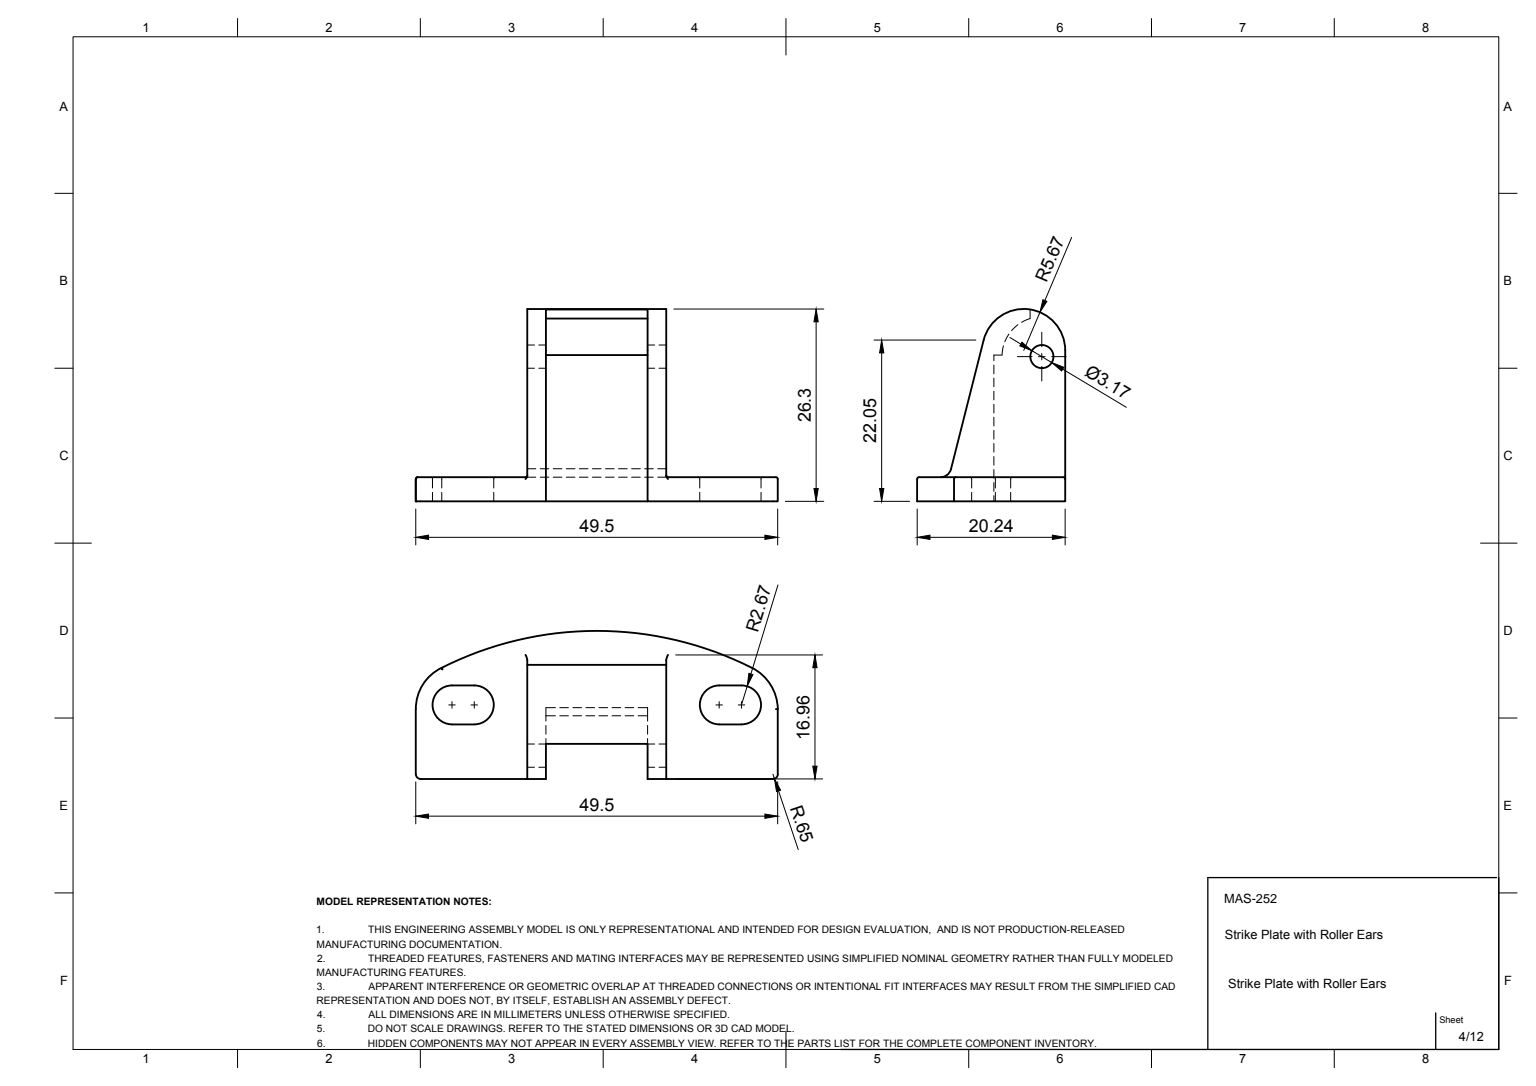
ISO-10303-21;
HEADER;
FILE_DESCRIPTION((''),'2;1');
FILE_NAME('Strike Plate with Roller Ears.step','2026-10-06T07:01:46+05:00',(''),(''),'','','');
FILE_SCHEMA (('AUTOMOTIVE_DESIGN { 1 0 10303 214 3 1 1 }'));
ENDSEC;
DATA;
#10=MECHANICAL_DESIGN_GEOMETRIC_PRESENTATION_REPRESENTATION('',(#139),#11396);
#109=SHAPE_REPRESENTATION_RELATIONSHIP('SRR','None',#11456,#124) ;
#124=ADVANCED_BREP_SHAPE_REPRESENTATION('',(#154),#11382) ;
#139=STYLED_ITEM('',(#11540),#154) ;
#154=MANIFOLD_SOLID_BREP('Strike Plate with Roller Ears',#5570) ;
#191=TOROIDAL_SURFACE('',#5927,0.5,0.25) ;
#192=TOROIDAL_SURFACE('',#5934,0.5,0.25) ;
#193=TOROIDAL_SURFACE('',#5944,2.915,0.25) ;
#194=TOROIDAL_SURFACE('',#5951,2.915,0.25) ;
#195=TOROIDAL_SURFACE('',#5967,2.915,0.25) ;
#196=TOROIDAL_SURFACE('',#5973,2.915,0.25) ;
#197=TOROIDAL_SURFACE('',#5982,5.95626157119474,0.25) ;
#198=TOROIDAL_SURFACE('',#5986,0.399999999999999,0.25) ;
#199=TOROIDAL_SURFACE('',#5990,6.2066222212067,0.25) ;
#200=TOROIDAL_SURFACE('',#5993,46.8573015873016,0.25) ;
#201=TOROIDAL_SURFACE('',#5997,0.400000000000004,0.25) ;
#264=B_SPLINE_CURVE_WITH_KNOTS('',3,(#9098,#9099,#9100,#9101,#9102,#9103,
#9104,#9105,#9106,#9107),.UNSPECIFIED.,.F.,.F.,(4,2,2,2,4),(0.129530190393873,
0.134403051839659,0.157131608255379,0.18177331440849,0.206415020561601),
 .UNSPECIFIED.) ;
#265=B_SPLINE_CURVE_WITH_KNOTS('',3,(#9118,#9119,#9120,#9121,#9122,#9123),
 .UNSPECIFIED.,.F.,.F.,(4,2,4),(0.126383060009627,0.145498866650295,0.174889571433522),
 .UNSPECIFIED.) ;
#266=B_SPLINE_CURVE_WITH_KNOTS('',3,(#9143,#9144,#9145,#9146,#9147,#9148),
 .UNSPECIFIED.,.F.,.F.,(4,2,4),(0.,0.029390704783227,0.0485065114238945),
 .UNSPECIFIED.) ;
#267=B_SPLINE_CURVE_WITH_KNOTS('',3,(#9157,#9158,#9159,#9160,#9161,#9162,
#9163,#9164,#9165,#9166),.UNSPECIFIED.,.F.,.F.,(4,2,2,2,4),(0.176028199507442,
0.200669905660553,0.225311611813664,0.248040168229384,0.252913029669695),
 .UNSPECIFIED.) ;
#268=B_SPLINE_CURVE_WITH_KNOTS('',3,(#9272,#9273,#9274,#9275,#9276,#9277,
#9278,#9279,#9280,#9281,#9282,#9283,#9284,#9285,#9286,#9287,#9288,#9289,
#9290,#9291,#9292,#9293,#9294,#9295,#9296,#9297,#9298,#9299),
 .UNSPECIFIED.,.F.,.F.,(4,3,3,3,3,3,3,3,3,4),(0.,0.196349541608207,0.38455924937953,
0.572733501937903,0.760877527668503,0.94899654600919,1.13718105053103,1.32530713430129,
1.51344881486777,1.57079633286566),.UNSPECIFIED.) ;
#269=B_SPLINE_CURVE_WITH_KNOTS('',3,(#9300,#9301,#9302,#9303,#9304,#9305,
#9306,#9307,#9308,#9309,#9310,#9311),.UNSPECIFIED.,.F.,.F.,(4,2,2,2,2,4),
(-0.0393939259354007,-0.0390590563554235,-0.0292978040547258,-0.0195312295441399,
-0.00976542256445868,0.),.UNSPECIFIED.) ;
#270=B_SPLINE_CURVE_WITH_KNOTS('',3,(#9327,#9328,#9329,#9330,#9331,#9332,
#9333,#9334,#9335,#9336,#9337,#9338),.UNSPECIFIED.,.F.,.F.,(4,2,2,2,2,4),
(-0.000371179043213308,0.,0.00972368624128075,0.0194900624985635,0.0292560287472632,
0.039021789210692),.UNSPECIFIED.) ;
#351=FACE_BOUND('',#949,.T.) ;
#352=FACE_BOUND('',#953,.T.) ;
#353=FACE_BOUND('',#961,.T.) ;
#354=FACE_BOUND('',#962,.T.) ;
#355=FACE_BOUND('',#992,.T.) ;
#356=FACE_BOUND('',#998,.T.) ;
#357=FACE_BOUND('',#1000,.T.) ;
#358=FACE_BOUND('',#1001,.T.) ;
#392=ELLIPSE('',#5926,0.353553390593277,0.25) ;
#393=ELLIPSE('',#5939,0.353553390593277,0.25) ;
#424=PLANE('',#5930) ;
#425=PLANE('',#5940) ;
#426=PLANE('',#5956) ;
#427=PLANE('',#5959) ;
#428=PLANE('',#5977) ;
#429=PLANE('',#6001) ;
#430=PLANE('',#6004) ;
#431=PLANE('',#6011) ;
#432=PLANE('',#6014) ;
#433=PLANE('',#6019) ;
#434=PLANE('',#6022) ;
#435=PLANE('',#6023) ;
#436=PLANE('',#6026) ;
#437=PLANE('',#6027) ;
#438=PLANE('',#6029) ;
#439=PLANE('',#6032) ;
#440=PLANE('',#6034) ;
#441=PLANE('',#6036) ;
#596=FACE_OUTER_BOUND('',#946,.T.) ;
#597=FACE_OUTER_BOUND('',#947,.T.) ;
#598=FACE_OUTER_BOUND('',#948,.T.) ;
#599=FACE_OUTER_BOUND('',#950,.T.) ;
#600=FACE_OUTER_BOUND('',#951,.T.) ;
#601=FACE_OUTER_BOUND('',#952,.T.) ;
#602=FACE_OUTER_BOUND('',#954,.T.) ;
#603=FACE_OUTER_BOUND('',#955,.T.) ;
#604=FACE_OUTER_BOUND('',#956,.T.) ;
#605=FACE_OUTER_BOUND('',#957,.T.) ;
#606=FACE_OUTER_BOUND('',#958,.T.) ;
#607=FACE_OUTER_BOUND('',#959,.T.) ;
#608=FACE_OUTER_BOUND('',#960,.T.) ;
#609=FACE_OUTER_BOUND('',#963,.T.) ;
#610=FACE_OUTER_BOUND('',#964,.T.) ;
#611=FACE_OUTER_BOUND('',#965,.T.) ;
#612=FACE_OUTER_BOUND('',#966,.T.) ;
#613=FACE_OUTER_BOUND('',#967,.T.) ;
#614=FACE_OUTER_BOUND('',#968,.T.) ;
#615=FACE_OUTER_BOUND('',#969,.T.) ;
#616=FACE_OUTER_BOUND('',#970,.T.) ;
#617=FACE_OUTER_BOUND('',#971,.T.) ;
#618=FACE_OUTER_BOUND('',#972,.T.) ;
#619=FACE_OUTER_BOUND('',#973,.T.) ;
#620=FACE_OUTER_BOUND('',#974,.T.) ;
#621=FACE_OUTER_BOUND('',#975,.T.) ;
#622=FACE_OUTER_BOUND('',#976,.T.) ;
#623=FACE_OUTER_BOUND('',#977,.T.) ;
#624=FACE_OUTER_BOUND('',#978,.T.) ;
#625=FACE_OUTER_BOUND('',#979,.T.) ;
#626=FACE_OUTER_BOUND('',#980,.T.) ;
#627=FACE_OUTER_BOUND('',#981,.T.) ;
#628=FACE_OUTER_BOUND('',#982,.T.) ;
#629=FACE_OUTER_BOUND('',#983,.T.) ;
#630=FACE_OUTER_BOUND('',#984,.T.) ;
#631=FACE_OUTER_BOUND('',#985,.T.) ;
#632=FACE_OUTER_BOUND('',#986,.T.) ;
#633=FACE_OUTER_BOUND('',#987,.T.) ;
#634=FACE_OUTER_BOUND('',#988,.T.) ;
#635=FACE_OUTER_BOUND('',#989,.T.) ;
#636=FACE_OUTER_BOUND('',#990,.T.) ;
#637=FACE_OUTER_BOUND('',#991,.T.) ;
#638=FACE_OUTER_BOUND('',#993,.T.) ;
#639=FACE_OUTER_BOUND('',#994,.T.) ;
#640=FACE_OUTER_BOUND('',#995,.T.) ;
#641=FACE_OUTER_BOUND('',#996,.T.) ;
#642=FACE_OUTER_BOUND('',#997,.T.) ;
#643=FACE_OUTER_BOUND('',#999,.T.) ;
#644=FACE_OUTER_BOUND('',#1002,.T.) ;
#645=FACE_OUTER_BOUND('',#1003,.T.) ;
#646=FACE_OUTER_BOUND('',#1004,.T.) ;
#647=FACE_OUTER_BOUND('',#1005,.T.) ;
#648=FACE_OUTER_BOUND('',#1006,.T.) ;
#649=FACE_OUTER_BOUND('',#1007,.T.) ;
#946=EDGE_LOOP('',(#3968,#3969,#3970,#3971,#3972)) ;
#947=EDGE_LOOP('',(#3973,#3974,#3975,#3976)) ;
#948=EDGE_LOOP('',(#3977,#3978,#3979,#3980,#3981,#3982)) ;
#949=EDGE_LOOP('',(#3983)) ;
#950=EDGE_LOOP('',(#3984,#3985,#3986,#3987)) ;
#951=EDGE_LOOP('',(#3988,#3989,#3990,#3991,#3992)) ;
#952=EDGE_LOOP('',(#3993,#3994,#3995,#3996,#3997,#3998)) ;
#953=EDGE_LOOP('',(#3999)) ;
#954=EDGE_LOOP('',(#4000,#4001,#4002,#4003)) ;
#955=EDGE_LOOP('',(#4004,#4005,#4006,#4007)) ;
#956=EDGE_LOOP('',(#4008,#4009,#4010,#4011)) ;
#957=EDGE_LOOP('',(#4012,#4013,#4014,#4015)) ;
#958=EDGE_LOOP('',(#4016,#4017,#4018,#4019)) ;
#959=EDGE_LOOP('',(#4020,#4021,#4022,#4023)) ;
#960=EDGE_LOOP('',(#4024,#4025,#4026,#4027,#4028,#4029,#4030,#4031,#4032,
#4033,#4034,#4035)) ;
#961=EDGE_LOOP('',(#4036,#4037,#4038,#4039)) ;
#962=EDGE_LOOP('',(#4040,#4041,#4042,#4043)) ;
#963=EDGE_LOOP('',(#4044,#4045,#4046,#4047)) ;
#964=EDGE_LOOP('',(#4048,#4049,#4050,#4051)) ;
#965=EDGE_LOOP('',(#4052,#4053,#4054,#4055)) ;
#966=EDGE_LOOP('',(#4056,#4057,#4058,#4059)) ;
#967=EDGE_LOOP('',(#4060,#4061,#4062,#4063)) ;
#968=EDGE_LOOP('',(#4064,#4065,#4066,#4067)) ;
#969=EDGE_LOOP('',(#4068,#4069,#4070,#4071)) ;
#970=EDGE_LOOP('',(#4072,#4073,#4074,#4075,#4076,#4077)) ;
#971=EDGE_LOOP('',(#4078,#4079,#4080,#4081)) ;
#972=EDGE_LOOP('',(#4082,#4083,#4084,#4085)) ;
#973=EDGE_LOOP('',(#4086,#4087,#4088,#4089)) ;
#974=EDGE_LOOP('',(#4090,#4091,#4092,#4093)) ;
#975=EDGE_LOOP('',(#4094,#4095,#4096,#4097)) ;
#976=EDGE_LOOP('',(#4098,#4099,#4100,#4101)) ;
#977=EDGE_LOOP('',(#4102,#4103,#4104,#4105)) ;
#978=EDGE_LOOP('',(#4106,#4107,#4108,#4109)) ;
#979=EDGE_LOOP('',(#4110,#4111,#4112,#4113)) ;
#980=EDGE_LOOP('',(#4114,#4115,#4116,#4117,#4118,#4119,#4120)) ;
#981=EDGE_LOOP('',(#4121,#4122,#4123,#4124)) ;
#982=EDGE_LOOP('',(#4125,#4126,#4127,#4128)) ;
#983=EDGE_LOOP('',(#4129,#4130,#4131,#4132)) ;
#984=EDGE_LOOP('',(#4133,#4134,#4135,#4136)) ;
#985=EDGE_LOOP('',(#4137,#4138,#4139,#4140)) ;
#986=EDGE_LOOP('',(#4141,#4142,#4143,#4144)) ;
#987=EDGE_LOOP('',(#4145,#4146,#4147,#4148)) ;
#988=EDGE_LOOP('',(#4149,#4150,#4151,#4152,#4153,#4154,#4155)) ;
#989=EDGE_LOOP('',(#4156,#4157,#4158,#4159)) ;
#990=EDGE_LOOP('',(#4160,#4161,#4162,#4163)) ;
#991=EDGE_LOOP('',(#4164,#4165,#4166,#4167,#4168,#4169,#4170)) ;
#992=EDGE_LOOP('',(#4171)) ;
#993=EDGE_LOOP('',(#4172,#4173,#4174,#4175)) ;
#994=EDGE_LOOP('',(#4176,#4177,#4178,#4179)) ;
#995=EDGE_LOOP('',(#4180,#4181,#4182,#4183)) ;
#996=EDGE_LOOP('',(#4184,#4185,#4186,#4187)) ;
#997=EDGE_LOOP('',(#4188,#4189,#4190,#4191,#4192,#4193,#4194)) ;
#998=EDGE_LOOP('',(#4195)) ;
#999=EDGE_LOOP('',(#4196,#4197,#4198,#4199,#4200,#4201,#4202,#4203,#4204,
#4205,#4206,#4207)) ;
#1000=EDGE_LOOP('',(#4208,#4209,#4210,#4211)) ;
#1001=EDGE_LOOP('',(#4212,#4213,#4214,#4215)) ;
#1002=EDGE_LOOP('',(#4216,#4217,#4218,#4219)) ;
#1003=EDGE_LOOP('',(#4220,#4221,#4222,#4223,#4224,#4225,#4226,#4227)) ;
#1004=EDGE_LOOP('',(#4228,#4229,#4230,#4231)) ;
#1005=EDGE_LOOP('',(#4232,#4233,#4234,#4235)) ;
#1006=EDGE_LOOP('',(#4236,#4237,#4238,#4239)) ;
#1007=EDGE_LOOP('',(#4240,#4241,#4242,#4243)) ;
#1326=LINE('',#9109,#1709) ;
#1327=LINE('',#9113,#1710) ;
#1328=LINE('',#9130,#1711) ;
#1329=LINE('',#9133,#1712) ;
#1330=LINE('',#9154,#1713) ;
#1331=LINE('',#9156,#1714) ;
#1332=LINE('',#9169,#1715) ;
#1333=LINE('',#9173,#1716) ;
#1334=LINE('',#9190,#1717) ;
#1335=LINE('',#9191,#1718) ;
#1336=LINE('',#9199,#1719) ;
#1337=LINE('',#9200,#1720) ;
#1338=LINE('',#9203,#1721) ;
#1339=LINE('',#9205,#1722) ;
#1340=LINE('',#9206,#1723) ;
#1341=LINE('',#9209,#1724) ;
#1342=LINE('',#9213,#1725) ;
#1343=LINE('',#9217,#1726) ;
#1344=LINE('',#9225,#1727) ;
#1345=LINE('',#9228,#1728) ;
#1346=LINE('',#9229,#1729) ;
#1347=LINE('',#9234,#1730) ;
#1348=LINE('',#9237,#1731) ;
#1349=LINE('',#9247,#1732) ;
#1350=LINE('',#9253,#1733) ;
#1351=LINE('',#9256,#1734) ;
#1352=LINE('',#9258,#1735) ;
#1353=LINE('',#9259,#1736) ;
#1354=LINE('',#9262,#1737) ;
#1355=LINE('',#9265,#1738) ;
#1356=LINE('',#9267,#1739) ;
#1357=LINE('',#9314,#1740) ;
#1358=LINE('',#9321,#1741) ;
#1359=LINE('',#9343,#1742) ;
#1360=LINE('',#9350,#1743) ;
#1361=LINE('',#9353,#1744) ;
#1362=LINE('',#9355,#1745) ;
#1363=LINE('',#9357,#1746) ;
#1364=LINE('',#9358,#1747) ;
#1365=LINE('',#9361,#1748) ;
#1366=LINE('',#9365,#1749) ;
#1367=LINE('',#9366,#1750) ;
#1368=LINE('',#9369,#1751) ;
#1369=LINE('',#9373,#1752) ;
#1370=LINE('',#9377,#1753) ;
#1371=LINE('',#9381,#1754) ;
#1372=LINE('',#9382,#1755) ;
#1373=LINE('',#9385,#1756) ;
#1374=LINE('',#9389,#1757) ;
#1375=LINE('',#9391,#1758) ;
#1376=LINE('',#9392,#1759) ;
#1377=LINE('',#9395,#1760) ;
#1378=LINE('',#9400,#1761) ;
#1379=LINE('',#9403,#1762) ;
#1380=LINE('',#9405,#1763) ;
#1381=LINE('',#9407,#1764) ;
#1382=LINE('',#9411,#1765) ;
#1383=LINE('',#9416,#1766) ;
#1384=LINE('',#9417,#1767) ;
#1385=LINE('',#9418,#1768) ;
#1386=LINE('',#9421,#1769) ;
#1387=LINE('',#9422,#1770) ;
#1388=LINE('',#9426,#1771) ;
#1389=LINE('',#9429,#1772) ;
#1390=LINE('',#9430,#1773) ;
#1391=LINE('',#9433,#1774) ;
#1392=LINE('',#9436,#1775) ;
#1393=LINE('',#9439,#1776) ;
#1394=LINE('',#9442,#1777) ;
#1395=LINE('',#9445,#1778) ;
#1396=LINE('',#9448,#1779) ;
#1709=VECTOR('',#6870,10.) ;
#1710=VECTOR('',#6873,10.) ;
#1711=VECTOR('',#6886,10.) ;
#1712=VECTOR('',#6889,10.) ;
#1713=VECTOR('',#6904,10.) ;
#1714=VECTOR('',#6905,10.) ;
#1715=VECTOR('',#6908,10.) ;
#1716=VECTOR('',#6911,10.) ;
#1717=VECTOR('',#6930,10.) ;
#1718=VECTOR('',#6931,10.) ;
#1719=VECTOR('',#6942,10.) ;
#1720=VECTOR('',#6943,10.) ;
#1721=VECTOR('',#6946,10.) ;
#1722=VECTOR('',#6947,10.) ;
#1723=VECTOR('',#6948,10.) ;
#1724=VECTOR('',#6951,10.) ;
#1725=VECTOR('',#6956,10.) ;
#1726=VECTOR('',#6959,10.) ;
#1727=VECTOR('',#6966,10.) ;
#1728=VECTOR('',#6969,10.) ;
#1729=VECTOR('',#6970,10.) ;
#1730=VECTOR('',#6973,10.) ;
#1731=VECTOR('',#6976,10.) ;
#1732=VECTOR('',#6989,10.) ;
#1733=VECTOR('',#6998,10.) ;
#1734=VECTOR('',#7001,10.) ;
#1735=VECTOR('',#7002,10.) ;
#1736=VECTOR('',#7003,10.) ;
#1737=VECTOR('',#7006,10.) ;
#1738=VECTOR('',#7011,10.) ;
#1739=VECTOR('',#7014,10.) ;
#1740=VECTOR('',#7021,10.) ;
#1741=VECTOR('',#7032,10.) ;
#1742=VECTOR('',#7045,10.) ;
#1743=VECTOR('',#7056,10.) ;
#1744=VECTOR('',#7059,10.) ;
#1745=VECTOR('',#7060,10.) ;
#1746=VECTOR('',#7061,10.) ;
#1747=VECTOR('',#7062,10.) ;
#1748=VECTOR('',#7065,10.) ;
#1749=VECTOR('',#7070,10.) ;
#1750=VECTOR('',#7071,10.) ;
#1751=VECTOR('',#7074,10.) ;
#1752=VECTOR('',#7079,10.) ;
#1753=VECTOR('',#7084,10.) ;
#1754=VECTOR('',#7089,10.) ;
#1755=VECTOR('',#7090,10.) ;
#1756=VECTOR('',#7093,10.) ;
#1757=VECTOR('',#7098,10.) ;
#1758=VECTOR('',#7099,10.) ;
#1759=VECTOR('',#7100,10.) ;
#1760=VECTOR('',#7103,1.585) ;
#1761=VECTOR('',#7110,1.585) ;
#1762=VECTOR('',#7113,10.) ;
#1763=VECTOR('',#7114,10.) ;
#1764=VECTOR('',#7115,10.) ;
#1765=VECTOR('',#7118,10.) ;
#1766=VECTOR('',#7123,10.) ;
#1767=VECTOR('',#7124,10.) ;
#1768=VECTOR('',#7125,10.) ;
#1769=VECTOR('',#7128,10.) ;
#1770=VECTOR('',#7129,10.) ;
#1771=VECTOR('',#7134,10.) ;
#1772=VECTOR('',#7137,10.) ;
#1773=VECTOR('',#7138,10.) ;
#1774=VECTOR('',#7143,10.) ;
#1775=VECTOR('',#7146,10.) ;
#1776=VECTOR('',#7149,10.) ;
#1777=VECTOR('',#7154,10.) ;
#1778=VECTOR('',#7159,10.) ;
#1779=VECTOR('',#7164,10.) ;
#2062=CIRCLE('',#5925,0.25) ;
#2063=CIRCLE('',#5928,0.25) ;
#2064=CIRCLE('',#5929,0.5) ;
#2065=CIRCLE('',#5931,1.48867477559092) ;
#2066=CIRCLE('',#5932,5.66550083849775) ;
#2067=CIRCLE('',#5933,1.585) ;
#2068=CIRCLE('',#5935,0.25) ;
#2069=CIRCLE('',#5936,0.25) ;
#2070=CIRCLE('',#5937,0.5) ;
#2071=CIRCLE('',#5941,5.66550083849775) ;
#2072=CIRCLE('',#5942,1.48867477559092) ;
#2073=CIRCLE('',#5943,1.585) ;
#2074=CIRCLE('',#5945,0.25) ;
#2075=CIRCLE('',#5946,2.665) ;
#2076=CIRCLE('',#5947,0.250000000000004) ;
#2077=CIRCLE('',#5948,2.915) ;
#2078=CIRCLE('',#5950,0.250000000000004) ;
#2079=CIRCLE('',#5952,0.250000000000004) ;
#2080=CIRCLE('',#5953,2.915) ;
#2081=CIRCLE('',#5954,2.665) ;
#2082=CIRCLE('',#5958,2.665) ;
#2083=CIRCLE('',#5960,0.400000000000004) ;
#2084=CIRCLE('',#5961,6.2066222212067) ;
#2085=CIRCLE('',#5962,46.8573015873016) ;
#2086=CIRCLE('',#5963,5.95626157119474) ;
#2087=CIRCLE('',#5964,0.399999999999999) ;
#2088=CIRCLE('',#5965,2.915) ;
#2089=CIRCLE('',#5966,2.915) ;
#2090=CIRCLE('',#5968,0.25) ;
#2091=CIRCLE('',#5969,2.665) ;
#2092=CIRCLE('',#5970,0.250000000000004) ;
#2093=CIRCLE('',#5972,0.250000000000004) ;
#2094=CIRCLE('',#5974,0.250000000000004) ;
#2095=CIRCLE('',#5975,2.665) ;
#2096=CIRCLE('',#5979,2.665) ;
#2097=CIRCLE('',#5983,6.20626157119474) ;
#2098=CIRCLE('',#5985,0.249999999999999) ;
#2099=CIRCLE('',#5987,0.250000000000004) ;
#2100=CIRCLE('',#5988,0.649999999999999) ;
#2101=CIRCLE('',#5991,6.4566222212067) ;
#2102=CIRCLE('',#5992,0.249999999999994) ;
#2103=CIRCLE('',#5994,47.1073015873016) ;
#2104=CIRCLE('',#5996,0.249999999999999) ;
#2105=CIRCLE('',#5998,0.249999999999999) ;
#2106=CIRCLE('',#5999,0.650000000000004) ;
#2107=CIRCLE('',#6003,0.649999999999999) ;
#2108=CIRCLE('',#6006,6.20626157119473) ;
#2109=CIRCLE('',#6008,47.1073015873016) ;
#2110=CIRCLE('',#6010,6.4566222212067) ;
#2111=CIRCLE('',#6013,0.650000000000004) ;
#2112=CIRCLE('',#6016,1.585) ;
#2113=CIRCLE('',#6018,1.585) ;
#2114=CIRCLE('',#6020,5.45) ;
#2115=CIRCLE('',#6021,5.66550083849775) ;
#2116=CIRCLE('',#6025,5.45) ;
#2117=CIRCLE('',#6028,5.66550083849775) ;
#2118=CIRCLE('',#6030,2.665) ;
#2119=CIRCLE('',#6031,2.665) ;
#2403=VERTEX_POINT('',#9096) ;
#2404=VERTEX_POINT('',#9097) ;
#2405=VERTEX_POINT('',#9108) ;
#2406=VERTEX_POINT('',#9110) ;
#2407=VERTEX_POINT('',#9112) ;
#2408=VERTEX_POINT('',#9116) ;
#2409=VERTEX_POINT('',#9117) ;
#2410=VERTEX_POINT('',#9127) ;
#2411=VERTEX_POINT('',#9129) ;
#2412=VERTEX_POINT('',#9131) ;
#2413=VERTEX_POINT('',#9134) ;
#2414=VERTEX_POINT('',#9137) ;
#2415=VERTEX_POINT('',#9138) ;
#2416=VERTEX_POINT('',#9140) ;
#2417=VERTEX_POINT('',#9142) ;
#2418=VERTEX_POINT('',#9151) ;
#2419=VERTEX_POINT('',#9152) ;
#2420=VERTEX_POINT('',#9155) ;
#2421=VERTEX_POINT('',#9168) ;
#2422=VERTEX_POINT('',#9170) ;
#2423=VERTEX_POINT('',#9172) ;
#2424=VERTEX_POINT('',#9175) ;
#2425=VERTEX_POINT('',#9178) ;
#2426=VERTEX_POINT('',#9179) ;
#2427=VERTEX_POINT('',#9181) ;
#2428=VERTEX_POINT('',#9183) ;
#2429=VERTEX_POINT('',#9187) ;
#2430=VERTEX_POINT('',#9188) ;
#2431=VERTEX_POINT('',#9193) ;
#2432=VERTEX_POINT('',#9194) ;
#2433=VERTEX_POINT('',#9202) ;
#2434=VERTEX_POINT('',#9204) ;
#2435=VERTEX_POINT('',#9208) ;
#2436=VERTEX_POINT('',#9212) ;
#2437=VERTEX_POINT('',#9214) ;
#2438=VERTEX_POINT('',#9216) ;
#2439=VERTEX_POINT('',#9218) ;
#2440=VERTEX_POINT('',#9220) ;
#2441=VERTEX_POINT('',#9222) ;
#2442=VERTEX_POINT('',#9224) ;
#2443=VERTEX_POINT('',#9226) ;
#2444=VERTEX_POINT('',#9230) ;
#2445=VERTEX_POINT('',#9231) ;
#2446=VERTEX_POINT('',#9233) ;
#2447=VERTEX_POINT('',#9235) ;
#2448=VERTEX_POINT('',#9239) ;
#2449=VERTEX_POINT('',#9241) ;
#2450=VERTEX_POINT('',#9245) ;
#2451=VERTEX_POINT('',#9249) ;
#2452=VERTEX_POINT('',#9255) ;
#2453=VERTEX_POINT('',#9257) ;
#2454=VERTEX_POINT('',#9261) ;
#2455=VERTEX_POINT('',#9269) ;
#2456=VERTEX_POINT('',#9270) ;
#2457=VERTEX_POINT('',#9313) ;
#2458=VERTEX_POINT('',#9317) ;
#2459=VERTEX_POINT('',#9323) ;
#2460=VERTEX_POINT('',#9324) ;
#2461=VERTEX_POINT('',#9342) ;
#2462=VERTEX_POINT('',#9346) ;
#2463=VERTEX_POINT('',#9352) ;
#2464=VERTEX_POINT('',#9354) ;
#2465=VERTEX_POINT('',#9356) ;
#2466=VERTEX_POINT('',#9360) ;
#2467=VERTEX_POINT('',#9364) ;
#2468=VERTEX_POINT('',#9368) ;
#2469=VERTEX_POINT('',#9372) ;
#2470=VERTEX_POINT('',#9376) ;
#2471=VERTEX_POINT('',#9380) ;
#2472=VERTEX_POINT('',#9384) ;
#2473=VERTEX_POINT('',#9388) ;
#2474=VERTEX_POINT('',#9390) ;
#2475=VERTEX_POINT('',#9394) ;
#2476=VERTEX_POINT('',#9398) ;
#2477=VERTEX_POINT('',#9402) ;
#2478=VERTEX_POINT('',#9404) ;
#2479=VERTEX_POINT('',#9406) ;
#2480=VERTEX_POINT('',#9408) ;
#2481=VERTEX_POINT('',#9410) ;
#2482=VERTEX_POINT('',#9414) ;
#2483=VERTEX_POINT('',#9415) ;
#2484=VERTEX_POINT('',#9420) ;
#2485=VERTEX_POINT('',#9424) ;
#2486=VERTEX_POINT('',#9428) ;
#2487=VERTEX_POINT('',#9435) ;
#2488=VERTEX_POINT('',#9438) ;
#2966=EDGE_CURVE('',#2403,#2404,#264,.T.) ;
#2967=EDGE_CURVE('',#2404,#2405,#1326,.T.) ;
#2968=EDGE_CURVE('',#2405,#2406,#2062,.T.) ;
#2969=EDGE_CURVE('',#2406,#2407,#1327,.T.) ;
#2970=EDGE_CURVE('',#2407,#2403,#392,.T.) ;
#2971=EDGE_CURVE('',#2408,#2409,#265,.T.) ;
#2972=EDGE_CURVE('',#2409,#2406,#2063,.T.) ;
#2973=EDGE_CURVE('',#2405,#2408,#2064,.T.) ;
#2974=EDGE_CURVE('',#2404,#2410,#2065,.T.) ;
#2975=EDGE_CURVE('',#2411,#2410,#1328,.T.) ;
#2976=EDGE_CURVE('',#2412,#2411,#2066,.T.) ;
#2977=EDGE_CURVE('',#2408,#2412,#1329,.T.) ;
#2978=EDGE_CURVE('',#2413,#2413,#2067,.T.) ;
#2979=EDGE_CURVE('',#2414,#2415,#2068,.T.) ;
#2980=EDGE_CURVE('',#2415,#2416,#2069,.T.) ;
#2981=EDGE_CURVE('',#2416,#2417,#266,.T.) ;
#2982=EDGE_CURVE('',#2417,#2414,#2070,.T.) ;
#2983=EDGE_CURVE('',#2418,#2419,#393,.F.) ;
#2984=EDGE_CURVE('',#2418,#2415,#1330,.T.) ;
#2985=EDGE_CURVE('',#2414,#2420,#1331,.T.) ;
#2986=EDGE_CURVE('',#2419,#2420,#267,.F.) ;
#2987=EDGE_CURVE('',#2417,#2421,#1332,.T.) ;
#2988=EDGE_CURVE('',#2421,#2422,#2071,.T.) ;
#2989=EDGE_CURVE('',#2422,#2423,#1333,.T.) ;
#2990=EDGE_CURVE('',#2423,#2420,#2072,.T.) ;
#2991=EDGE_CURVE('',#2424,#2424,#2073,.T.) ;
#2992=EDGE_CURVE('',#2425,#2426,#2074,.T.) ;
#2993=EDGE_CURVE('',#2426,#2427,#2075,.T.) ;
#2994=EDGE_CURVE('',#2427,#2428,#2076,.T.) ;
#2995=EDGE_CURVE('',#2428,#2425,#2077,.T.) ;
#2996=EDGE_CURVE('',#2429,#2430,#2078,.T.) ;
#2997=EDGE_CURVE('',#2430,#2428,#1334,.T.) ;
#2998=EDGE_CURVE('',#2427,#2429,#1335,.T.) ;
#2999=EDGE_CURVE('',#2431,#2432,#2079,.T.) ;
#3000=EDGE_CURVE('',#2432,#2430,#2080,.T.) ;
#3001=EDGE_CURVE('',#2429,#2431,#2081,.T.) ;
#3002=EDGE_CURVE('',#2425,#2432,#1336,.T.) ;
#3003=EDGE_CURVE('',#2431,#2426,#1337,.T.) ;
#3004=EDGE_CURVE('',#2433,#2427,#1338,.T.) ;
#3005=EDGE_CURVE('',#2433,#2434,#1339,.T.) ;
#3006=EDGE_CURVE('',#2434,#2429,#1340,.T.) ;
#3007=EDGE_CURVE('',#2435,#2426,#1341,.T.) ;
#3008=EDGE_CURVE('',#2435,#2433,#2082,.T.) ;
#3009=EDGE_CURVE('',#2436,#2406,#1342,.T.) ;
#3010=EDGE_CURVE('',#2437,#2436,#2083,.T.) ;
#3011=EDGE_CURVE('',#2438,#2437,#1343,.T.) ;
#3012=EDGE_CURVE('',#2439,#2438,#2084,.T.) ;
#3013=EDGE_CURVE('',#2440,#2439,#2085,.T.) ;
#3014=EDGE_CURVE('',#2441,#2440,#2086,.T.) ;
#3015=EDGE_CURVE('',#2442,#2441,#1344,.T.) ;
#3016=EDGE_CURVE('',#2443,#2442,#2087,.T.) ;
#3017=EDGE_CURVE('',#2415,#2443,#1345,.T.) ;
#3018=EDGE_CURVE('',#2407,#2418,#1346,.T.) ;
#3019=EDGE_CURVE('',#2444,#2445,#2088,.T.) ;
#3020=EDGE_CURVE('',#2446,#2444,#1347,.T.) ;
#3021=EDGE_CURVE('',#2447,#2446,#2089,.T.) ;
#3022=EDGE_CURVE('',#2445,#2447,#1348,.T.) ;
#3023=EDGE_CURVE('',#2445,#2448,#2090,.T.) ;
#3024=EDGE_CURVE('',#2448,#2449,#2091,.T.) ;
#3025=EDGE_CURVE('',#2449,#2444,#2092,.T.) ;
#3026=EDGE_CURVE('',#2450,#2446,#2093,.T.) ;
#3027=EDGE_CURVE('',#2449,#2450,#1349,.T.) ;
#3028=EDGE_CURVE('',#2451,#2447,#2094,.T.) ;
#3029=EDGE_CURVE('',#2450,#2451,#2095,.T.) ;
#3030=EDGE_CURVE('',#2451,#2448,#1350,.T.) ;
#3031=EDGE_CURVE('',#2452,#2449,#1351,.T.) ;
#3032=EDGE_CURVE('',#2452,#2453,#1352,.T.) ;
#3033=EDGE_CURVE('',#2453,#2450,#1353,.T.) ;
#3034=EDGE_CURVE('',#2454,#2448,#1354,.T.) ;
#3035=EDGE_CURVE('',#2454,#2452,#2096,.T.) ;
#3036=EDGE_CURVE('',#2419,#2403,#1355,.T.) ;
#3037=EDGE_CURVE('',#2410,#2423,#1356,.T.) ;
#3038=EDGE_CURVE('',#2455,#2456,#2097,.T.) ;
#3039=EDGE_CURVE('',#2456,#2441,#268,.T.) ;
#3040=EDGE_CURVE('',#2440,#2455,#269,.T.) ;
#3041=EDGE_CURVE('',#2456,#2457,#1357,.T.) ;
#3042=EDGE_CURVE('',#2457,#2442,#2098,.T.) ;
#3043=EDGE_CURVE('',#2458,#2443,#2099,.T.) ;
#3044=EDGE_CURVE('',#2457,#2458,#2100,.T.) ;
#3045=EDGE_CURVE('',#2458,#2416,#1358,.T.) ;
#3046=EDGE_CURVE('',#2459,#2460,#2101,.T.) ;
#3047=EDGE_CURVE('',#2460,#2439,#2102,.T.) ;
#3048=EDGE_CURVE('',#2438,#2459,#270,.T.) ;
#3049=EDGE_CURVE('',#2460,#2455,#2103,.T.) ;
#3050=EDGE_CURVE('',#2409,#2461,#1359,.T.) ;
#3051=EDGE_CURVE('',#2461,#2436,#2104,.T.) ;
#3052=EDGE_CURVE('',#2462,#2437,#2105,.T.) ;
#3053=EDGE_CURVE('',#2461,#2462,#2106,.T.) ;
#3054=EDGE_CURVE('',#2462,#2459,#1360,.T.) ;
#3055=EDGE_CURVE('',#2463,#2458,#1361,.T.) ;
#3056=EDGE_CURVE('',#2464,#2463,#1362,.T.) ;
#3057=EDGE_CURVE('',#2464,#2465,#1363,.T.) ;
#3058=EDGE_CURVE('',#2465,#2421,#1364,.T.) ;
#3059=EDGE_CURVE('',#2466,#2457,#1365,.T.) ;
#3060=EDGE_CURVE('',#2466,#2463,#2107,.T.) ;
#3061=EDGE_CURVE('',#2467,#2456,#1366,.T.) ;
#3062=EDGE_CURVE('',#2466,#2467,#1367,.T.) ;
#3063=EDGE_CURVE('',#2468,#2455,#1368,.T.) ;
#3064=EDGE_CURVE('',#2468,#2467,#2108,.T.) ;
#3065=EDGE_CURVE('',#2469,#2460,#1369,.T.) ;
#3066=EDGE_CURVE('',#2469,#2468,#2109,.T.) ;
#3067=EDGE_CURVE('',#2470,#2459,#1370,.T.) ;
#3068=EDGE_CURVE('',#2470,#2469,#2110,.T.) ;
#3069=EDGE_CURVE('',#2471,#2462,#1371,.T.) ;
#3070=EDGE_CURVE('',#2470,#2471,#1372,.T.) ;
#3071=EDGE_CURVE('',#2472,#2461,#1373,.T.) ;
#3072=EDGE_CURVE('',#2472,#2471,#2111,.T.) ;
#3073=EDGE_CURVE('',#2412,#2473,#1374,.T.) ;
#3074=EDGE_CURVE('',#2473,#2474,#1375,.T.) ;
#3075=EDGE_CURVE('',#2472,#2474,#1376,.T.) ;
#3076=EDGE_CURVE('',#2413,#2475,#1377,.T.) ;
#3077=EDGE_CURVE('',#2475,#2475,#2112,.T.) ;
#3078=EDGE_CURVE('',#2476,#2476,#2113,.T.) ;
#3079=EDGE_CURVE('',#2476,#2424,#1378,.T.) ;
#3080=EDGE_CURVE('',#2477,#2464,#1379,.T.) ;
#3081=EDGE_CURVE('',#2478,#2477,#1380,.T.) ;
#3082=EDGE_CURVE('',#2479,#2478,#1381,.T.) ;
#3083=EDGE_CURVE('',#2480,#2479,#2114,.T.) ;
#3084=EDGE_CURVE('',#2481,#2480,#1382,.T.) ;
#3085=EDGE_CURVE('',#2465,#2481,#2115,.T.) ;
#3086=EDGE_CURVE('',#2482,#2483,#1383,.T.) ;
#3087=EDGE_CURVE('',#2482,#2478,#1384,.T.) ;
#3088=EDGE_CURVE('',#2483,#2477,#1385,.T.) ;
#3089=EDGE_CURVE('',#2484,#2482,#1386,.T.) ;
#3090=EDGE_CURVE('',#2484,#2479,#1387,.T.) ;
#3091=EDGE_CURVE('',#2485,#2484,#2116,.T.) ;
#3092=EDGE_CURVE('',#2485,#2480,#1388,.T.) ;
#3093=EDGE_CURVE('',#2481,#2486,#1389,.T.) ;
#3094=EDGE_CURVE('',#2486,#2485,#1390,.T.) ;
#3095=EDGE_CURVE('',#2486,#2473,#2117,.T.) ;
#3096=EDGE_CURVE('',#2474,#2483,#1391,.T.) ;
#3097=EDGE_CURVE('',#2487,#2454,#1392,.T.) ;
#3098=EDGE_CURVE('',#2453,#2487,#2118,.T.) ;
#3099=EDGE_CURVE('',#2488,#2435,#1393,.T.) ;
#3100=EDGE_CURVE('',#2434,#2488,#2119,.T.) ;
#3101=EDGE_CURVE('',#2411,#2422,#1394,.T.) ;
#3102=EDGE_CURVE('',#2487,#2451,#1395,.T.) ;
#3103=EDGE_CURVE('',#2488,#2431,#1396,.T.) ;
#3968=ORIENTED_EDGE('',*,*,#2966,.T.) ;
#3969=ORIENTED_EDGE('',*,*,#2967,.T.) ;
#3970=ORIENTED_EDGE('',*,*,#2968,.T.) ;
#3971=ORIENTED_EDGE('',*,*,#2969,.T.) ;
#3972=ORIENTED_EDGE('',*,*,#2970,.T.) ;
#3973=ORIENTED_EDGE('',*,*,#2971,.T.) ;
#3974=ORIENTED_EDGE('',*,*,#2972,.T.) ;
#3975=ORIENTED_EDGE('',*,*,#2968,.F.) ;
#3976=ORIENTED_EDGE('',*,*,#2973,.T.) ;
#3977=ORIENTED_EDGE('',*,*,#2973,.F.) ;
#3978=ORIENTED_EDGE('',*,*,#2967,.F.) ;
#3979=ORIENTED_EDGE('',*,*,#2974,.T.) ;
#3980=ORIENTED_EDGE('',*,*,#2975,.F.) ;
#3981=ORIENTED_EDGE('',*,*,#2976,.F.) ;
#3982=ORIENTED_EDGE('',*,*,#2977,.F.) ;
#3983=ORIENTED_EDGE('',*,*,#2978,.T.) ;
#3984=ORIENTED_EDGE('',*,*,#2979,.T.) ;
#3985=ORIENTED_EDGE('',*,*,#2980,.T.) ;
#3986=ORIENTED_EDGE('',*,*,#2981,.T.) ;
#3987=ORIENTED_EDGE('',*,*,#2982,.T.) ;
#3988=ORIENTED_EDGE('',*,*,#2983,.F.) ;
#3989=ORIENTED_EDGE('',*,*,#2984,.T.) ;
#3990=ORIENTED_EDGE('',*,*,#2979,.F.) ;
#3991=ORIENTED_EDGE('',*,*,#2985,.T.) ;
#3992=ORIENTED_EDGE('',*,*,#2986,.F.) ;
#3993=ORIENTED_EDGE('',*,*,#2985,.F.) ;
#3994=ORIENTED_EDGE('',*,*,#2982,.F.) ;
#3995=ORIENTED_EDGE('',*,*,#2987,.T.) ;
#3996=ORIENTED_EDGE('',*,*,#2988,.T.) ;
#3997=ORIENTED_EDGE('',*,*,#2989,.T.) ;
#3998=ORIENTED_EDGE('',*,*,#2990,.T.) ;
#3999=ORIENTED_EDGE('',*,*,#2991,.T.) ;
#4000=ORIENTED_EDGE('',*,*,#2992,.T.) ;
#4001=ORIENTED_EDGE('',*,*,#2993,.T.) ;
#4002=ORIENTED_EDGE('',*,*,#2994,.T.) ;
#4003=ORIENTED_EDGE('',*,*,#2995,.T.) ;
#4004=ORIENTED_EDGE('',*,*,#2996,.T.) ;
#4005=ORIENTED_EDGE('',*,*,#2997,.T.) ;
#4006=ORIENTED_EDGE('',*,*,#2994,.F.) ;
#4007=ORIENTED_EDGE('',*,*,#2998,.T.) ;
#4008=ORIENTED_EDGE('',*,*,#2999,.T.) ;
#4009=ORIENTED_EDGE('',*,*,#3000,.T.) ;
#4010=ORIENTED_EDGE('',*,*,#2996,.F.) ;
#4011=ORIENTED_EDGE('',*,*,#3001,.T.) ;
#4012=ORIENTED_EDGE('',*,*,#2992,.F.) ;
#4013=ORIENTED_EDGE('',*,*,#3002,.T.) ;
#4014=ORIENTED_EDGE('',*,*,#2999,.F.) ;
#4015=ORIENTED_EDGE('',*,*,#3003,.T.) ;
#4016=ORIENTED_EDGE('',*,*,#2998,.F.) ;
#4017=ORIENTED_EDGE('',*,*,#3004,.F.) ;
#4018=ORIENTED_EDGE('',*,*,#3005,.T.) ;
#4019=ORIENTED_EDGE('',*,*,#3006,.T.) ;
#4020=ORIENTED_EDGE('',*,*,#2993,.F.) ;
#4021=ORIENTED_EDGE('',*,*,#3007,.F.) ;
#4022=ORIENTED_EDGE('',*,*,#3008,.T.) ;
#4023=ORIENTED_EDGE('',*,*,#3004,.T.) ;
#4024=ORIENTED_EDGE('',*,*,#2969,.F.) ;
#4025=ORIENTED_EDGE('',*,*,#3009,.F.) ;
#4026=ORIENTED_EDGE('',*,*,#3010,.F.) ;
#4027=ORIENTED_EDGE('',*,*,#3011,.F.) ;
#4028=ORIENTED_EDGE('',*,*,#3012,.F.) ;
#4029=ORIENTED_EDGE('',*,*,#3013,.F.) ;
#4030=ORIENTED_EDGE('',*,*,#3014,.F.) ;
#4031=ORIENTED_EDGE('',*,*,#3015,.F.) ;
#4032=ORIENTED_EDGE('',*,*,#3016,.F.) ;
#4033=ORIENTED_EDGE('',*,*,#3017,.F.) ;
#4034=ORIENTED_EDGE('',*,*,#2984,.F.) ;
#4035=ORIENTED_EDGE('',*,*,#3018,.F.) ;
#4036=ORIENTED_EDGE('',*,*,#3019,.F.) ;
#4037=ORIENTED_EDGE('',*,*,#3020,.F.) ;
#4038=ORIENTED_EDGE('',*,*,#3021,.F.) ;
#4039=ORIENTED_EDGE('',*,*,#3022,.F.) ;
#4040=ORIENTED_EDGE('',*,*,#2995,.F.) ;
#4041=ORIENTED_EDGE('',*,*,#2997,.F.) ;
#4042=ORIENTED_EDGE('',*,*,#3000,.F.) ;
#4043=ORIENTED_EDGE('',*,*,#3002,.F.) ;
#4044=ORIENTED_EDGE('',*,*,#3023,.T.) ;
#4045=ORIENTED_EDGE('',*,*,#3024,.T.) ;
#4046=ORIENTED_EDGE('',*,*,#3025,.T.) ;
#4047=ORIENTED_EDGE('',*,*,#3019,.T.) ;
#4048=ORIENTED_EDGE('',*,*,#3026,.T.) ;
#4049=ORIENTED_EDGE('',*,*,#3020,.T.) ;
#4050=ORIENTED_EDGE('',*,*,#3025,.F.) ;
#4051=ORIENTED_EDGE('',*,*,#3027,.T.) ;
#4052=ORIENTED_EDGE('',*,*,#3028,.T.) ;
#4053=ORIENTED_EDGE('',*,*,#3021,.T.) ;
#4054=ORIENTED_EDGE('',*,*,#3026,.F.) ;
#4055=ORIENTED_EDGE('',*,*,#3029,.T.) ;
#4056=ORIENTED_EDGE('',*,*,#3023,.F.) ;
#4057=ORIENTED_EDGE('',*,*,#3022,.T.) ;
#4058=ORIENTED_EDGE('',*,*,#3028,.F.) ;
#4059=ORIENTED_EDGE('',*,*,#3030,.T.) ;
#4060=ORIENTED_EDGE('',*,*,#3027,.F.) ;
#4061=ORIENTED_EDGE('',*,*,#3031,.F.) ;
#4062=ORIENTED_EDGE('',*,*,#3032,.T.) ;
#4063=ORIENTED_EDGE('',*,*,#3033,.T.) ;
#4064=ORIENTED_EDGE('',*,*,#3024,.F.) ;
#4065=ORIENTED_EDGE('',*,*,#3034,.F.) ;
#4066=ORIENTED_EDGE('',*,*,#3035,.T.) ;
#4067=ORIENTED_EDGE('',*,*,#3031,.T.) ;
#4068=ORIENTED_EDGE('',*,*,#3036,.T.) ;
#4069=ORIENTED_EDGE('',*,*,#2970,.F.) ;
#4070=ORIENTED_EDGE('',*,*,#3018,.T.) ;
#4071=ORIENTED_EDGE('',*,*,#2983,.T.) ;
#4072=ORIENTED_EDGE('',*,*,#3036,.F.) ;
#4073=ORIENTED_EDGE('',*,*,#2986,.T.) ;
#4074=ORIENTED_EDGE('',*,*,#2990,.F.) ;
#4075=ORIENTED_EDGE('',*,*,#3037,.F.) ;
#4076=ORIENTED_EDGE('',*,*,#2974,.F.) ;
#4077=ORIENTED_EDGE('',*,*,#2966,.F.) ;
#4078=ORIENTED_EDGE('',*,*,#3038,.T.) ;
#4079=ORIENTED_EDGE('',*,*,#3039,.T.) ;
#4080=ORIENTED_EDGE('',*,*,#3014,.T.) ;
#4081=ORIENTED_EDGE('',*,*,#3040,.T.) ;
#4082=ORIENTED_EDGE('',*,*,#3039,.F.) ;
#4083=ORIENTED_EDGE('',*,*,#3041,.T.) ;
#4084=ORIENTED_EDGE('',*,*,#3042,.T.) ;
#4085=ORIENTED_EDGE('',*,*,#3015,.T.) ;
#4086=ORIENTED_EDGE('',*,*,#3043,.T.) ;
#4087=ORIENTED_EDGE('',*,*,#3016,.T.) ;
#4088=ORIENTED_EDGE('',*,*,#3042,.F.) ;
#4089=ORIENTED_EDGE('',*,*,#3044,.T.) ;
#4090=ORIENTED_EDGE('',*,*,#2980,.F.) ;
#4091=ORIENTED_EDGE('',*,*,#3017,.T.) ;
#4092=ORIENTED_EDGE('',*,*,#3043,.F.) ;
#4093=ORIENTED_EDGE('',*,*,#3045,.T.) ;
#4094=ORIENTED_EDGE('',*,*,#3046,.T.) ;
#4095=ORIENTED_EDGE('',*,*,#3047,.T.) ;
#4096=ORIENTED_EDGE('',*,*,#3012,.T.) ;
#4097=ORIENTED_EDGE('',*,*,#3048,.T.) ;
#4098=ORIENTED_EDGE('',*,*,#3013,.T.) ;
#4099=ORIENTED_EDGE('',*,*,#3047,.F.) ;
#4100=ORIENTED_EDGE('',*,*,#3049,.T.) ;
#4101=ORIENTED_EDGE('',*,*,#3040,.F.) ;
#4102=ORIENTED_EDGE('',*,*,#2972,.F.) ;
#4103=ORIENTED_EDGE('',*,*,#3050,.T.) ;
#4104=ORIENTED_EDGE('',*,*,#3051,.T.) ;
#4105=ORIENTED_EDGE('',*,*,#3009,.T.) ;
#4106=ORIENTED_EDGE('',*,*,#3052,.T.) ;
#4107=ORIENTED_EDGE('',*,*,#3010,.T.) ;
#4108=ORIENTED_EDGE('',*,*,#3051,.F.) ;
#4109=ORIENTED_EDGE('',*,*,#3053,.T.) ;
#4110=ORIENTED_EDGE('',*,*,#3011,.T.) ;
#4111=ORIENTED_EDGE('',*,*,#3052,.F.) ;
#4112=ORIENTED_EDGE('',*,*,#3054,.T.) ;
#4113=ORIENTED_EDGE('',*,*,#3048,.F.) ;
#4114=ORIENTED_EDGE('',*,*,#2981,.F.) ;
#4115=ORIENTED_EDGE('',*,*,#3045,.F.) ;
#4116=ORIENTED_EDGE('',*,*,#3055,.F.) ;
#4117=ORIENTED_EDGE('',*,*,#3056,.F.) ;
#4118=ORIENTED_EDGE('',*,*,#3057,.T.) ;
#4119=ORIENTED_EDGE('',*,*,#3058,.T.) ;
#4120=ORIENTED_EDGE('',*,*,#2987,.F.) ;
#4121=ORIENTED_EDGE('',*,*,#3044,.F.) ;
#4122=ORIENTED_EDGE('',*,*,#3059,.F.) ;
#4123=ORIENTED_EDGE('',*,*,#3060,.T.) ;
#4124=ORIENTED_EDGE('',*,*,#3055,.T.) ;
#4125=ORIENTED_EDGE('',*,*,#3041,.F.) ;
#4126=ORIENTED_EDGE('',*,*,#3061,.F.) ;
#4127=ORIENTED_EDGE('',*,*,#3062,.F.) ;
#4128=ORIENTED_EDGE('',*,*,#3059,.T.) ;
#4129=ORIENTED_EDGE('',*,*,#3038,.F.) ;
#4130=ORIENTED_EDGE('',*,*,#3063,.F.) ;
#4131=ORIENTED_EDGE('',*,*,#3064,.T.) ;
#4132=ORIENTED_EDGE('',*,*,#3061,.T.) ;
#4133=ORIENTED_EDGE('',*,*,#3049,.F.) ;
#4134=ORIENTED_EDGE('',*,*,#3065,.F.) ;
#4135=ORIENTED_EDGE('',*,*,#3066,.T.) ;
#4136=ORIENTED_EDGE('',*,*,#3063,.T.) ;
#4137=ORIENTED_EDGE('',*,*,#3046,.F.) ;
#4138=ORIENTED_EDGE('',*,*,#3067,.F.) ;
#4139=ORIENTED_EDGE('',*,*,#3068,.T.) ;
#4140=ORIENTED_EDGE('',*,*,#3065,.T.) ;
#4141=ORIENTED_EDGE('',*,*,#3054,.F.) ;
#4142=ORIENTED_EDGE('',*,*,#3069,.F.) ;
#4143=ORIENTED_EDGE('',*,*,#3070,.F.) ;
#4144=ORIENTED_EDGE('',*,*,#3067,.T.) ;
#4145=ORIENTED_EDGE('',*,*,#3053,.F.) ;
#4146=ORIENTED_EDGE('',*,*,#3071,.F.) ;
#4147=ORIENTED_EDGE('',*,*,#3072,.T.) ;
#4148=ORIENTED_EDGE('',*,*,#3069,.T.) ;
#4149=ORIENTED_EDGE('',*,*,#2977,.T.) ;
#4150=ORIENTED_EDGE('',*,*,#3073,.T.) ;
#4151=ORIENTED_EDGE('',*,*,#3074,.T.) ;
#4152=ORIENTED_EDGE('',*,*,#3075,.F.) ;
#4153=ORIENTED_EDGE('',*,*,#3071,.T.) ;
#4154=ORIENTED_EDGE('',*,*,#3050,.F.) ;
#4155=ORIENTED_EDGE('',*,*,#2971,.F.) ;
#4156=ORIENTED_EDGE('',*,*,#2978,.F.) ;
#4157=ORIENTED_EDGE('',*,*,#3076,.T.) ;
#4158=ORIENTED_EDGE('',*,*,#3077,.F.) ;
#4159=ORIENTED_EDGE('',*,*,#3076,.F.) ;
#4160=ORIENTED_EDGE('',*,*,#3078,.F.) ;
#4161=ORIENTED_EDGE('',*,*,#3079,.T.) ;
#4162=ORIENTED_EDGE('',*,*,#2991,.F.) ;
#4163=ORIENTED_EDGE('',*,*,#3079,.F.) ;
#4164=ORIENTED_EDGE('',*,*,#3057,.F.) ;
#4165=ORIENTED_EDGE('',*,*,#3080,.F.) ;
#4166=ORIENTED_EDGE('',*,*,#3081,.F.) ;
#4167=ORIENTED_EDGE('',*,*,#3082,.F.) ;
#4168=ORIENTED_EDGE('',*,*,#3083,.F.) ;
#4169=ORIENTED_EDGE('',*,*,#3084,.F.) ;
#4170=ORIENTED_EDGE('',*,*,#3085,.F.) ;
#4171=ORIENTED_EDGE('',*,*,#3078,.T.) ;
#4172=ORIENTED_EDGE('',*,*,#3086,.F.) ;
#4173=ORIENTED_EDGE('',*,*,#3087,.T.) ;
#4174=ORIENTED_EDGE('',*,*,#3081,.T.) ;
#4175=ORIENTED_EDGE('',*,*,#3088,.F.) ;
#4176=ORIENTED_EDGE('',*,*,#3089,.F.) ;
#4177=ORIENTED_EDGE('',*,*,#3090,.T.) ;
#4178=ORIENTED_EDGE('',*,*,#3082,.T.) ;
#4179=ORIENTED_EDGE('',*,*,#3087,.F.) ;
#4180=ORIENTED_EDGE('',*,*,#3091,.F.) ;
#4181=ORIENTED_EDGE('',*,*,#3092,.T.) ;
#4182=ORIENTED_EDGE('',*,*,#3083,.T.) ;
#4183=ORIENTED_EDGE('',*,*,#3090,.F.) ;
#4184=ORIENTED_EDGE('',*,*,#3093,.F.) ;
#4185=ORIENTED_EDGE('',*,*,#3084,.T.) ;
#4186=ORIENTED_EDGE('',*,*,#3092,.F.) ;
#4187=ORIENTED_EDGE('',*,*,#3094,.F.) ;
#4188=ORIENTED_EDGE('',*,*,#3074,.F.) ;
#4189=ORIENTED_EDGE('',*,*,#3095,.F.) ;
#4190=ORIENTED_EDGE('',*,*,#3094,.T.) ;
#4191=ORIENTED_EDGE('',*,*,#3091,.T.) ;
#4192=ORIENTED_EDGE('',*,*,#3089,.T.) ;
#4193=ORIENTED_EDGE('',*,*,#3086,.T.) ;
#4194=ORIENTED_EDGE('',*,*,#3096,.F.) ;
#4195=ORIENTED_EDGE('',*,*,#3077,.T.) ;
#4196=ORIENTED_EDGE('',*,*,#3096,.T.) ;
#4197=ORIENTED_EDGE('',*,*,#3088,.T.) ;
#4198=ORIENTED_EDGE('',*,*,#3080,.T.) ;
#4199=ORIENTED_EDGE('',*,*,#3056,.T.) ;
#4200=ORIENTED_EDGE('',*,*,#3060,.F.) ;
#4201=ORIENTED_EDGE('',*,*,#3062,.T.) ;
#4202=ORIENTED_EDGE('',*,*,#3064,.F.) ;
#4203=ORIENTED_EDGE('',*,*,#3066,.F.) ;
#4204=ORIENTED_EDGE('',*,*,#3068,.F.) ;
#4205=ORIENTED_EDGE('',*,*,#3070,.T.) ;
#4206=ORIENTED_EDGE('',*,*,#3072,.F.) ;
#4207=ORIENTED_EDGE('',*,*,#3075,.T.) ;
#4208=ORIENTED_EDGE('',*,*,#3035,.F.) ;
#4209=ORIENTED_EDGE('',*,*,#3097,.F.) ;
#4210=ORIENTED_EDGE('',*,*,#3098,.F.) ;
#4211=ORIENTED_EDGE('',*,*,#3032,.F.) ;
#4212=ORIENTED_EDGE('',*,*,#3008,.F.) ;
#4213=ORIENTED_EDGE('',*,*,#3099,.F.) ;
#4214=ORIENTED_EDGE('',*,*,#3100,.F.) ;
#4215=ORIENTED_EDGE('',*,*,#3005,.F.) ;
#4216=ORIENTED_EDGE('',*,*,#2975,.T.) ;
#4217=ORIENTED_EDGE('',*,*,#3037,.T.) ;
#4218=ORIENTED_EDGE('',*,*,#2989,.F.) ;
#4219=ORIENTED_EDGE('',*,*,#3101,.F.) ;
#4220=ORIENTED_EDGE('',*,*,#3095,.T.) ;
#4221=ORIENTED_EDGE('',*,*,#3073,.F.) ;
#4222=ORIENTED_EDGE('',*,*,#2976,.T.) ;
#4223=ORIENTED_EDGE('',*,*,#3101,.T.) ;
#4224=ORIENTED_EDGE('',*,*,#2988,.F.) ;
#4225=ORIENTED_EDGE('',*,*,#3058,.F.) ;
#4226=ORIENTED_EDGE('',*,*,#3085,.T.) ;
#4227=ORIENTED_EDGE('',*,*,#3093,.T.) ;
#4228=ORIENTED_EDGE('',*,*,#3030,.F.) ;
#4229=ORIENTED_EDGE('',*,*,#3102,.F.) ;
#4230=ORIENTED_EDGE('',*,*,#3097,.T.) ;
#4231=ORIENTED_EDGE('',*,*,#3034,.T.) ;
#4232=ORIENTED_EDGE('',*,*,#3029,.F.) ;
#4233=ORIENTED_EDGE('',*,*,#3033,.F.) ;
#4234=ORIENTED_EDGE('',*,*,#3098,.T.) ;
#4235=ORIENTED_EDGE('',*,*,#3102,.T.) ;
#4236=ORIENTED_EDGE('',*,*,#3003,.F.) ;
#4237=ORIENTED_EDGE('',*,*,#3103,.F.) ;
#4238=ORIENTED_EDGE('',*,*,#3099,.T.) ;
#4239=ORIENTED_EDGE('',*,*,#3007,.T.) ;
#4240=ORIENTED_EDGE('',*,*,#3001,.F.) ;
#4241=ORIENTED_EDGE('',*,*,#3006,.F.) ;
#4242=ORIENTED_EDGE('',*,*,#3100,.T.) ;
#4243=ORIENTED_EDGE('',*,*,#3103,.T.) ;
#5129=CYLINDRICAL_SURFACE('',#5924,0.25) ;
#5130=CYLINDRICAL_SURFACE('',#5938,0.25) ;
#5131=CYLINDRICAL_SURFACE('',#5949,0.25) ;
#5132=CYLINDRICAL_SURFACE('',#5955,0.25) ;
#5133=CYLINDRICAL_SURFACE('',#5957,2.665) ;
#5134=CYLINDRICAL_SURFACE('',#5971,0.25) ;
#5135=CYLINDRICAL_SURFACE('',#5976,0.25) ;
#5136=CYLINDRICAL_SURFACE('',#5978,2.665) ;
#5137=CYLINDRICAL_SURFACE('',#5980,0.25) ;
#5138=CYLINDRICAL_SURFACE('',#5981,1.48867477559092) ;
#5139=CYLINDRICAL_SURFACE('',#5984,0.25) ;
#5140=CYLINDRICAL_SURFACE('',#5989,0.25) ;
#5141=CYLINDRICAL_SURFACE('',#5995,0.25) ;
#5142=CYLINDRICAL_SURFACE('',#6000,0.25) ;
#5143=CYLINDRICAL_SURFACE('',#6002,0.649999999999999) ;
#5144=CYLINDRICAL_SURFACE('',#6005,6.20626157119473) ;
#5145=CYLINDRICAL_SURFACE('',#6007,47.1073015873016) ;
#5146=CYLINDRICAL_SURFACE('',#6009,6.4566222212067) ;
#5147=CYLINDRICAL_SURFACE('',#6012,0.650000000000004) ;
#5148=CYLINDRICAL_SURFACE('',#6015,1.585) ;
#5149=CYLINDRICAL_SURFACE('',#6017,1.585) ;
#5150=CYLINDRICAL_SURFACE('',#6024,5.45) ;
#5151=CYLINDRICAL_SURFACE('',#6033,5.66550083849775) ;
#5152=CYLINDRICAL_SURFACE('',#6035,2.665) ;
#5153=CYLINDRICAL_SURFACE('',#6037,2.665) ;
#5321=ADVANCED_FACE('',(#596),#5129,.F.) ;
#5322=ADVANCED_FACE('',(#597),#191,.F.) ;
#5323=ADVANCED_FACE('',(#598,#351),#424,.F.) ;
#5324=ADVANCED_FACE('',(#599),#192,.F.) ;
#5325=ADVANCED_FACE('',(#600),#5130,.F.) ;
#5326=ADVANCED_FACE('',(#601,#352),#425,.T.) ;
#5327=ADVANCED_FACE('',(#602),#193,.T.) ;
#5328=ADVANCED_FACE('',(#603),#5131,.T.) ;
#5329=ADVANCED_FACE('',(#604),#194,.T.) ;
#5330=ADVANCED_FACE('',(#605),#5132,.T.) ;
#5331=ADVANCED_FACE('',(#606),#426,.T.) ;
#5332=ADVANCED_FACE('',(#607),#5133,.F.) ;
#5333=ADVANCED_FACE('',(#608,#353,#354),#427,.T.) ;
#5334=ADVANCED_FACE('',(#609),#195,.T.) ;
#5335=ADVANCED_FACE('',(#610),#5134,.T.) ;
#5336=ADVANCED_FACE('',(#611),#196,.T.) ;
#5337=ADVANCED_FACE('',(#612),#5135,.T.) ;
#5338=ADVANCED_FACE('',(#613),#428,.T.) ;
#5339=ADVANCED_FACE('',(#614),#5136,.F.) ;
#5340=ADVANCED_FACE('',(#615),#5137,.F.) ;
#5341=ADVANCED_FACE('',(#616),#5138,.F.) ;
#5342=ADVANCED_FACE('',(#617),#197,.T.) ;
#5343=ADVANCED_FACE('',(#618),#5139,.T.) ;
#5344=ADVANCED_FACE('',(#619),#198,.T.) ;
#5345=ADVANCED_FACE('',(#620),#5140,.T.) ;
#5346=ADVANCED_FACE('',(#621),#199,.T.) ;
#5347=ADVANCED_FACE('',(#622),#200,.T.) ;
#5348=ADVANCED_FACE('',(#623),#5141,.T.) ;
#5349=ADVANCED_FACE('',(#624),#201,.T.) ;
#5350=ADVANCED_FACE('',(#625),#5142,.T.) ;
#5351=ADVANCED_FACE('',(#626),#429,.T.) ;
#5352=ADVANCED_FACE('',(#627),#5143,.T.) ;
#5353=ADVANCED_FACE('',(#628),#430,.T.) ;
#5354=ADVANCED_FACE('',(#629),#5144,.T.) ;
#5355=ADVANCED_FACE('',(#630),#5145,.T.) ;
#5356=ADVANCED_FACE('',(#631),#5146,.T.) ;
#5357=ADVANCED_FACE('',(#632),#431,.T.) ;
#5358=ADVANCED_FACE('',(#633),#5147,.T.) ;
#5359=ADVANCED_FACE('',(#634),#432,.T.) ;
#5360=ADVANCED_FACE('',(#635),#5148,.F.) ;
#5361=ADVANCED_FACE('',(#636),#5149,.F.) ;
#5362=ADVANCED_FACE('',(#637,#355),#433,.F.) ;
#5363=ADVANCED_FACE('',(#638),#434,.F.) ;
#5364=ADVANCED_FACE('',(#639),#435,.F.) ;
#5365=ADVANCED_FACE('',(#640),#5150,.F.) ;
#5366=ADVANCED_FACE('',(#641),#436,.F.) ;
#5367=ADVANCED_FACE('',(#642,#356),#437,.T.) ;
#5368=ADVANCED_FACE('',(#643,#357,#358),#438,.F.) ;
#5369=ADVANCED_FACE('',(#644),#439,.T.) ;
#5370=ADVANCED_FACE('',(#645),#5151,.T.) ;
#5371=ADVANCED_FACE('',(#646),#440,.T.) ;
#5372=ADVANCED_FACE('',(#647),#5152,.F.) ;
#5373=ADVANCED_FACE('',(#648),#441,.T.) ;
#5374=ADVANCED_FACE('',(#649),#5153,.F.) ;
#5570=CLOSED_SHELL('',(#5321,#5322,#5323,#5324,#5325,#5326,#5327,#5328,
#5329,#5330,#5331,#5332,#5333,#5334,#5335,#5336,#5337,#5338,#5339,#5340,
#5341,#5342,#5343,#5344,#5345,#5346,#5347,#5348,#5349,#5350,#5351,#5352,
#5353,#5354,#5355,#5356,#5357,#5358,#5359,#5360,#5361,#5362,#5363,#5364,
#5365,#5366,#5367,#5368,#5369,#5370,#5371,#5372,#5373,#5374)) ;
#5923=AXIS2_PLACEMENT_3D('',#9094,#6866,#6867) ;
#5924=AXIS2_PLACEMENT_3D('',#9095,#6868,#6869) ;
#5925=AXIS2_PLACEMENT_3D('',#9111,#6871,#6872) ;
#5926=AXIS2_PLACEMENT_3D('',#9114,#6874,#6875) ;
#5927=AXIS2_PLACEMENT_3D('',#9115,#6876,#6877) ;
#5928=AXIS2_PLACEMENT_3D('',#9124,#6878,#6879) ;
#5929=AXIS2_PLACEMENT_3D('',#9125,#6880,#6881) ;
#5930=AXIS2_PLACEMENT_3D('',#9126,#6882,#6883) ;
#5931=AXIS2_PLACEMENT_3D('',#9128,#6884,#6885) ;
#5932=AXIS2_PLACEMENT_3D('',#9132,#6887,#6888) ;
#5933=AXIS2_PLACEMENT_3D('',#9135,#6890,#6891) ;
#5934=AXIS2_PLACEMENT_3D('',#9136,#6892,#6893) ;
#5935=AXIS2_PLACEMENT_3D('',#9139,#6894,#6895) ;
#5936=AXIS2_PLACEMENT_3D('',#9141,#6896,#6897) ;
#5937=AXIS2_PLACEMENT_3D('',#9149,#6898,#6899) ;
#5938=AXIS2_PLACEMENT_3D('',#9150,#6900,#6901) ;
#5939=AXIS2_PLACEMENT_3D('',#9153,#6902,#6903) ;
#5940=AXIS2_PLACEMENT_3D('',#9167,#6906,#6907) ;
#5941=AXIS2_PLACEMENT_3D('',#9171,#6909,#6910) ;
#5942=AXIS2_PLACEMENT_3D('',#9174,#6912,#6913) ;
#5943=AXIS2_PLACEMENT_3D('',#9176,#6914,#6915) ;
#5944=AXIS2_PLACEMENT_3D('',#9177,#6916,#6917) ;
#5945=AXIS2_PLACEMENT_3D('',#9180,#6918,#6919) ;
#5946=AXIS2_PLACEMENT_3D('',#9182,#6920,#6921) ;
#5947=AXIS2_PLACEMENT_3D('',#9184,#6922,#6923) ;
#5948=AXIS2_PLACEMENT_3D('',#9185,#6924,#6925) ;
#5949=AXIS2_PLACEMENT_3D('',#9186,#6926,#6927) ;
#5950=AXIS2_PLACEMENT_3D('',#9189,#6928,#6929) ;
#5951=AXIS2_PLACEMENT_3D('',#9192,#6932,#6933) ;
#5952=AXIS2_PLACEMENT_3D('',#9195,#6934,#6935) ;
#5953=AXIS2_PLACEMENT_3D('',#9196,#6936,#6937) ;
#5954=AXIS2_PLACEMENT_3D('',#9197,#6938,#6939) ;
#5955=AXIS2_PLACEMENT_3D('',#9198,#6940,#6941) ;
#5956=AXIS2_PLACEMENT_3D('',#9201,#6944,#6945) ;
#5957=AXIS2_PLACEMENT_3D('',#9207,#6949,#6950) ;
#5958=AXIS2_PLACEMENT_3D('',#9210,#6952,#6953) ;
#5959=AXIS2_PLACEMENT_3D('',#9211,#6954,#6955) ;
#5960=AXIS2_PLACEMENT_3D('',#9215,#6957,#6958) ;
#5961=AXIS2_PLACEMENT_3D('',#9219,#6960,#6961) ;
#5962=AXIS2_PLACEMENT_3D('',#9221,#6962,#6963) ;
#5963=AXIS2_PLACEMENT_3D('',#9223,#6964,#6965) ;
#5964=AXIS2_PLACEMENT_3D('',#9227,#6967,#6968) ;
#5965=AXIS2_PLACEMENT_3D('',#9232,#6971,#6972) ;
#5966=AXIS2_PLACEMENT_3D('',#9236,#6974,#6975) ;
#5967=AXIS2_PLACEMENT_3D('',#9238,#6977,#6978) ;
#5968=AXIS2_PLACEMENT_3D('',#9240,#6979,#6980) ;
#5969=AXIS2_PLACEMENT_3D('',#9242,#6981,#6982) ;
#5970=AXIS2_PLACEMENT_3D('',#9243,#6983,#6984) ;
#5971=AXIS2_PLACEMENT_3D('',#9244,#6985,#6986) ;
#5972=AXIS2_PLACEMENT_3D('',#9246,#6987,#6988) ;
#5973=AXIS2_PLACEMENT_3D('',#9248,#6990,#6991) ;
#5974=AXIS2_PLACEMENT_3D('',#9250,#6992,#6993) ;
#5975=AXIS2_PLACEMENT_3D('',#9251,#6994,#6995) ;
#5976=AXIS2_PLACEMENT_3D('',#9252,#6996,#6997) ;
#5977=AXIS2_PLACEMENT_3D('',#9254,#6999,#7000) ;
#5978=AXIS2_PLACEMENT_3D('',#9260,#7004,#7005) ;
#5979=AXIS2_PLACEMENT_3D('',#9263,#7007,#7008) ;
#5980=AXIS2_PLACEMENT_3D('',#9264,#7009,#7010) ;
#5981=AXIS2_PLACEMENT_3D('',#9266,#7012,#7013) ;
#5982=AXIS2_PLACEMENT_3D('',#9268,#7015,#7016) ;
#5983=AXIS2_PLACEMENT_3D('',#9271,#7017,#7018) ;
#5984=AXIS2_PLACEMENT_3D('',#9312,#7019,#7020) ;
#5985=AXIS2_PLACEMENT_3D('',#9315,#7022,#7023) ;
#5986=AXIS2_PLACEMENT_3D('',#9316,#7024,#7025) ;
#5987=AXIS2_PLACEMENT_3D('',#9318,#7026,#7027) ;
#5988=AXIS2_PLACEMENT_3D('',#9319,#7028,#7029) ;
#5989=AXIS2_PLACEMENT_3D('',#9320,#7030,#7031) ;
#5990=AXIS2_PLACEMENT_3D('',#9322,#7033,#7034) ;
#5991=AXIS2_PLACEMENT_3D('',#9325,#7035,#7036) ;
#5992=AXIS2_PLACEMENT_3D('',#9326,#7037,#7038) ;
#5993=AXIS2_PLACEMENT_3D('',#9339,#7039,#7040) ;
#5994=AXIS2_PLACEMENT_3D('',#9340,#7041,#7042) ;
#5995=AXIS2_PLACEMENT_3D('',#9341,#7043,#7044) ;
#5996=AXIS2_PLACEMENT_3D('',#9344,#7046,#7047) ;
#5997=AXIS2_PLACEMENT_3D('',#9345,#7048,#7049) ;
#5998=AXIS2_PLACEMENT_3D('',#9347,#7050,#7051) ;
#5999=AXIS2_PLACEMENT_3D('',#9348,#7052,#7053) ;
#6000=AXIS2_PLACEMENT_3D('',#9349,#7054,#7055) ;
#6001=AXIS2_PLACEMENT_3D('',#9351,#7057,#7058) ;
#6002=AXIS2_PLACEMENT_3D('',#9359,#7063,#7064) ;
#6003=AXIS2_PLACEMENT_3D('',#9362,#7066,#7067) ;
#6004=AXIS2_PLACEMENT_3D('',#9363,#7068,#7069) ;
#6005=AXIS2_PLACEMENT_3D('',#9367,#7072,#7073) ;
#6006=AXIS2_PLACEMENT_3D('',#9370,#7075,#7076) ;
#6007=AXIS2_PLACEMENT_3D('',#9371,#7077,#7078) ;
#6008=AXIS2_PLACEMENT_3D('',#9374,#7080,#7081) ;
#6009=AXIS2_PLACEMENT_3D('',#9375,#7082,#7083) ;
#6010=AXIS2_PLACEMENT_3D('',#9378,#7085,#7086) ;
#6011=AXIS2_PLACEMENT_3D('',#9379,#7087,#7088) ;
#6012=AXIS2_PLACEMENT_3D('',#9383,#7091,#7092) ;
#6013=AXIS2_PLACEMENT_3D('',#9386,#7094,#7095) ;
#6014=AXIS2_PLACEMENT_3D('',#9387,#7096,#7097) ;
#6015=AXIS2_PLACEMENT_3D('',#9393,#7101,#7102) ;
#6016=AXIS2_PLACEMENT_3D('',#9396,#7104,#7105) ;
#6017=AXIS2_PLACEMENT_3D('',#9397,#7106,#7107) ;
#6018=AXIS2_PLACEMENT_3D('',#9399,#7108,#7109) ;
#6019=AXIS2_PLACEMENT_3D('',#9401,#7111,#7112) ;
#6020=AXIS2_PLACEMENT_3D('',#9409,#7116,#7117) ;
#6021=AXIS2_PLACEMENT_3D('',#9412,#7119,#7120) ;
#6022=AXIS2_PLACEMENT_3D('',#9413,#7121,#7122) ;
#6023=AXIS2_PLACEMENT_3D('',#9419,#7126,#7127) ;
#6024=AXIS2_PLACEMENT_3D('',#9423,#7130,#7131) ;
#6025=AXIS2_PLACEMENT_3D('',#9425,#7132,#7133) ;
#6026=AXIS2_PLACEMENT_3D('',#9427,#7135,#7136) ;
#6027=AXIS2_PLACEMENT_3D('',#9431,#7139,#7140) ;
#6028=AXIS2_PLACEMENT_3D('',#9432,#7141,#7142) ;
#6029=AXIS2_PLACEMENT_3D('',#9434,#7144,#7145) ;
#6030=AXIS2_PLACEMENT_3D('',#9437,#7147,#7148) ;
#6031=AXIS2_PLACEMENT_3D('',#9440,#7150,#7151) ;
#6032=AXIS2_PLACEMENT_3D('',#9441,#7152,#7153) ;
#6033=AXIS2_PLACEMENT_3D('',#9443,#7155,#7156) ;
#6034=AXIS2_PLACEMENT_3D('',#9444,#7157,#7158) ;
#6035=AXIS2_PLACEMENT_3D('',#9446,#7160,#7161) ;
#6036=AXIS2_PLACEMENT_3D('',#9447,#7162,#7163) ;
#6037=AXIS2_PLACEMENT_3D('',#9449,#7165,#7166) ;
#6866=DIRECTION('axis',(0.,0.,1.)) ;
#6867=DIRECTION('refdir',(1.,0.,0.)) ;
#6868=DIRECTION('center_axis',(0.,0.,-1.)) ;
#6869=DIRECTION('ref_axis',(0.707106781186548,-0.707106781186548,0.)) ;
#6870=DIRECTION('',(0.,0.,-1.)) ;
#6871=DIRECTION('center_axis',(0.,0.,-1.)) ;
#6872=DIRECTION('ref_axis',(1.,0.,0.)) ;
#6873=DIRECTION('',(0.,0.,1.)) ;
#6874=DIRECTION('center_axis',(0.707106781186554,0.,0.707106781186541)) ;
#6875=DIRECTION('ref_axis',(0.707106781186541,0.,-0.707106781186554)) ;
#6876=DIRECTION('center_axis',(-1.,0.,0.)) ;
#6877=DIRECTION('ref_axis',(0.,0.,1.)) ;
#6878=DIRECTION('center_axis',(1.,0.,0.)) ;
#6879=DIRECTION('ref_axis',(0.,0.707106781186548,-0.707106781186548)) ;
#6880=DIRECTION('center_axis',(-1.,0.,0.)) ;
#6881=DIRECTION('ref_axis',(0.,0.707106781186548,-0.707106781186548)) ;
#6882=DIRECTION('center_axis',(1.,0.,0.)) ;
#6883=DIRECTION('ref_axis',(0.,0.,-1.)) ;
#6884=DIRECTION('center_axis',(1.,0.,0.)) ;
#6885=DIRECTION('ref_axis',(0.,-0.997759953305869,0.0668960057034024)) ;
#6886=DIRECTION('',(0.,-0.969490981460344,0.245126981107871)) ;
#6887=DIRECTION('center_axis',(1.,0.,0.)) ;
#6888=DIRECTION('ref_axis',(0.,0.00361481447269016,-0.999993466536821)) ;
#6889=DIRECTION('',(0.,1.,0.)) ;
#6890=DIRECTION('center_axis',(1.,0.,0.)) ;
#6891=DIRECTION('ref_axis',(0.,0.,-1.)) ;
#6892=DIRECTION('center_axis',(1.,0.,0.)) ;
#6893=DIRECTION('ref_axis',(0.,0.,-1.)) ;
#6894=DIRECTION('center_axis',(0.,0.,1.)) ;
#6895=DIRECTION('ref_axis',(-1.,0.,0.)) ;
#6896=DIRECTION('center_axis',(-1.,0.,0.)) ;
#6897=DIRECTION('ref_axis',(0.,0.707106781186548,-0.707106781186548)) ;
#6898=DIRECTION('center_axis',(1.,0.,0.)) ;
#6899=DIRECTION('ref_axis',(0.,0.707106781186548,-0.707106781186548)) ;
#6900=DIRECTION('center_axis',(0.,0.,1.)) ;
#6901=DIRECTION('ref_axis',(-0.707106781186548,-0.707106781186548,0.)) ;
#6902=DIRECTION('center_axis',(-0.707106781186554,0.,0.707106781186541)) ;
#6903=DIRECTION('ref_axis',(-0.707106781186541,0.,-0.707106781186554)) ;
#6904=DIRECTION('',(0.,0.,-1.)) ;
#6905=DIRECTION('',(0.,0.,1.)) ;
#6906=DIRECTION('center_axis',(1.,0.,0.)) ;
#6907=DIRECTION('ref_axis',(0.,0.,-1.)) ;
#6908=DIRECTION('',(0.,1.,0.)) ;
#6909=DIRECTION('center_axis',(1.,0.,0.)) ;
#6910=DIRECTION('ref_axis',(0.,0.00361481447269016,-0.999993466536821)) ;
#6911=DIRECTION('',(0.,-0.969490981460344,0.245126981107871)) ;
#6912=DIRECTION('center_axis',(-1.,0.,0.)) ;
#6913=DIRECTION('ref_axis',(0.,-0.997759953305869,0.0668960057034024)) ;
#6914=DIRECTION('center_axis',(-1.,0.,0.)) ;
#6915=DIRECTION('ref_axis',(0.,0.,-1.)) ;
#6916=DIRECTION('center_axis',(0.,-1.,0.)) ;
#6917=DIRECTION('ref_axis',(0.,0.,-1.)) ;
#6918=DIRECTION('center_axis',(-1.,0.,0.)) ;
#6919=DIRECTION('ref_axis',(0.,1.,0.)) ;
#6920=DIRECTION('center_axis',(0.,-1.,0.)) ;
#6921=DIRECTION('ref_axis',(-1.,0.,0.)) ;
#6922=DIRECTION('center_axis',(-1.,0.,0.)) ;
#6923=DIRECTION('ref_axis',(0.,0.,1.)) ;
#6924=DIRECTION('center_axis',(0.,1.,0.)) ;
#6925=DIRECTION('ref_axis',(-1.,0.,0.)) ;
#6926=DIRECTION('center_axis',(1.,0.,0.)) ;
#6927=DIRECTION('ref_axis',(0.,0.707106781186543,0.707106781186552)) ;
#6928=DIRECTION('center_axis',(-1.,0.,0.)) ;
#6929=DIRECTION('ref_axis',(0.,0.,1.)) ;
#6930=DIRECTION('',(-1.,0.,0.)) ;
#6931=DIRECTION('',(1.,0.,0.)) ;
#6932=DIRECTION('center_axis',(0.,-1.,0.)) ;
#6933=DIRECTION('ref_axis',(0.,0.,-1.)) ;
#6934=DIRECTION('center_axis',(1.,0.,0.)) ;
#6935=DIRECTION('ref_axis',(0.,0.,-1.)) ;
#6936=DIRECTION('center_axis',(0.,1.,0.)) ;
#6937=DIRECTION('ref_axis',(1.,0.,0.)) ;
#6938=DIRECTION('center_axis',(0.,-1.,0.)) ;
#6939=DIRECTION('ref_axis',(1.,0.,0.)) ;
#6940=DIRECTION('center_axis',(-1.,0.,0.)) ;
#6941=DIRECTION('ref_axis',(0.,0.707106781186543,-0.707106781186552)) ;
#6942=DIRECTION('',(1.,0.,0.)) ;
#6943=DIRECTION('',(-1.,0.,0.)) ;
#6944=DIRECTION('center_axis',(0.,0.,1.)) ;
#6945=DIRECTION('ref_axis',(1.,0.,0.)) ;
#6946=DIRECTION('',(0.,1.,0.)) ;
#6947=DIRECTION('',(1.,0.,0.)) ;
#6948=DIRECTION('',(0.,1.,0.)) ;
#6949=DIRECTION('center_axis',(0.,1.,0.)) ;
#6950=DIRECTION('ref_axis',(-8.33188010975728E-16,0.,-1.)) ;
#6951=DIRECTION('',(0.,1.,0.)) ;
#6952=DIRECTION('center_axis',(0.,-1.,0.)) ;
#6953=DIRECTION('ref_axis',(-8.33188010975728E-16,0.,-1.)) ;
#6954=DIRECTION('center_axis',(0.,1.,0.)) ;
#6955=DIRECTION('ref_axis',(1.,0.,0.)) ;
#6956=DIRECTION('',(1.,0.,0.)) ;
#6957=DIRECTION('center_axis',(0.,-1.,0.)) ;
#6958=DIRECTION('ref_axis',(-0.707106781186544,0.,-0.707106781186551)) ;
#6959=DIRECTION('',(0.,0.,-1.)) ;
#6960=DIRECTION('center_axis',(0.,-1.,0.)) ;
#6961=DIRECTION('ref_axis',(-0.846732995614247,0.,0.532018076890367)) ;
#6962=DIRECTION('center_axis',(0.,-1.,0.)) ;
#6963=DIRECTION('ref_axis',(4.71359210659789E-17,0.,1.)) ;
#6964=DIRECTION('center_axis',(0.,-1.,0.)) ;
#6965=DIRECTION('ref_axis',(0.846732995614246,0.,0.532018076890367)) ;
#6966=DIRECTION('',(0.,0.,1.)) ;
#6967=DIRECTION('center_axis',(0.,-1.,0.)) ;
#6968=DIRECTION('ref_axis',(0.707106781186544,0.,-0.707106781186551)) ;
#6969=DIRECTION('',(1.,0.,0.)) ;
#6970=DIRECTION('',(1.,0.,0.)) ;
#6971=DIRECTION('center_axis',(0.,1.,0.)) ;
#6972=DIRECTION('ref_axis',(-1.,0.,0.)) ;
#6973=DIRECTION('',(-1.,0.,0.)) ;
#6974=DIRECTION('center_axis',(0.,1.,0.)) ;
#6975=DIRECTION('ref_axis',(1.,0.,0.)) ;
#6976=DIRECTION('',(1.,0.,0.)) ;
#6977=DIRECTION('center_axis',(0.,-1.,0.)) ;
#6978=DIRECTION('ref_axis',(0.,0.,-1.)) ;
#6979=DIRECTION('center_axis',(-1.,0.,0.)) ;
#6980=DIRECTION('ref_axis',(0.,1.,0.)) ;
#6981=DIRECTION('center_axis',(0.,-1.,0.)) ;
#6982=DIRECTION('ref_axis',(-1.,0.,0.)) ;
#6983=DIRECTION('center_axis',(-1.,0.,0.)) ;
#6984=DIRECTION('ref_axis',(0.,0.,1.)) ;
#6985=DIRECTION('center_axis',(1.,0.,0.)) ;
#6986=DIRECTION('ref_axis',(0.,0.707106781186543,0.707106781186552)) ;
#6987=DIRECTION('center_axis',(-1.,0.,-8.88178419700113E-15)) ;
#6988=DIRECTION('ref_axis',(-8.88178419700113E-15,0.,1.)) ;
#6989=DIRECTION('',(1.,0.,0.)) ;
#6990=DIRECTION('center_axis',(0.,-1.,0.)) ;
#6991=DIRECTION('ref_axis',(0.,0.,-1.)) ;
#6992=DIRECTION('center_axis',(1.,0.,0.)) ;
#6993=DIRECTION('ref_axis',(0.,0.,-1.)) ;
#6994=DIRECTION('center_axis',(0.,-1.,0.)) ;
#6995=DIRECTION('ref_axis',(1.,0.,0.)) ;
#6996=DIRECTION('center_axis',(-1.,0.,0.)) ;
#6997=DIRECTION('ref_axis',(0.,0.707106781186543,-0.707106781186552)) ;
#6998=DIRECTION('',(-1.,0.,0.)) ;
#6999=DIRECTION('center_axis',(0.,0.,1.)) ;
#7000=DIRECTION('ref_axis',(1.,0.,0.)) ;
#7001=DIRECTION('',(0.,1.,0.)) ;
#7002=DIRECTION('',(1.,0.,0.)) ;
#7003=DIRECTION('',(0.,1.,0.)) ;
#7004=DIRECTION('center_axis',(0.,1.,0.)) ;
#7005=DIRECTION('ref_axis',(-8.33188010975728E-16,0.,-1.)) ;
#7006=DIRECTION('',(0.,1.,0.)) ;
#7007=DIRECTION('center_axis',(0.,-1.,0.)) ;
#7008=DIRECTION('ref_axis',(-8.33188010975728E-16,0.,-1.)) ;
#7009=DIRECTION('center_axis',(-1.,0.,0.)) ;
#7010=DIRECTION('ref_axis',(0.,-0.99932673530985,-0.0366889096997627)) ;
#7011=DIRECTION('',(-1.,0.,0.)) ;
#7012=DIRECTION('center_axis',(1.,0.,0.)) ;
#7013=DIRECTION('ref_axis',(0.,-0.997759953305869,0.0668960057034024)) ;
#7014=DIRECTION('',(1.,0.,0.)) ;
#7015=DIRECTION('center_axis',(0.,1.,0.)) ;
#7016=DIRECTION('ref_axis',(0.,0.,1.)) ;
#7017=DIRECTION('center_axis',(0.,1.,0.)) ;
#7018=DIRECTION('ref_axis',(0.846732995614246,0.,0.532018076890367)) ;
#7019=DIRECTION('center_axis',(0.,0.,-1.)) ;
#7020=DIRECTION('ref_axis',(0.707106781186552,0.707106781186543,0.)) ;
#7021=DIRECTION('',(0.,0.,-1.)) ;
#7022=DIRECTION('center_axis',(0.,0.,1.)) ;
#7023=DIRECTION('ref_axis',(1.,0.,0.)) ;
#7024=DIRECTION('center_axis',(0.,1.,0.)) ;
#7025=DIRECTION('ref_axis',(0.,0.,1.)) ;
#7026=DIRECTION('center_axis',(1.,0.,0.)) ;
#7027=DIRECTION('ref_axis',(0.,0.,-1.)) ;
#7028=DIRECTION('center_axis',(0.,1.,0.)) ;
#7029=DIRECTION('ref_axis',(0.707106781186544,0.,-0.707106781186551)) ;
#7030=DIRECTION('center_axis',(-1.,0.,0.)) ;
#7031=DIRECTION('ref_axis',(0.,0.707106781186555,-0.70710678118654)) ;
#7032=DIRECTION('',(-1.,0.,0.)) ;
#7033=DIRECTION('center_axis',(0.,1.,0.)) ;
#7034=DIRECTION('ref_axis',(0.,0.,1.)) ;
#7035=DIRECTION('center_axis',(0.,1.,0.)) ;
#7036=DIRECTION('ref_axis',(-0.846732995614247,0.,0.532018076890367)) ;
#7037=DIRECTION('center_axis',(-0.893020597138892,0.,-0.450015792040343)) ;
#7038=DIRECTION('ref_axis',(-0.450015792040343,0.,0.893020597138892)) ;
#7039=DIRECTION('center_axis',(0.,1.,0.)) ;
#7040=DIRECTION('ref_axis',(0.,0.,1.)) ;
#7041=DIRECTION('center_axis',(0.,1.,0.)) ;
#7042=DIRECTION('ref_axis',(4.71359210659789E-17,0.,1.)) ;
#7043=DIRECTION('center_axis',(-1.,0.,0.)) ;
#7044=DIRECTION('ref_axis',(0.,0.707106781186555,-0.70710678118654)) ;
#7045=DIRECTION('',(-1.,0.,0.)) ;
#7046=DIRECTION('center_axis',(1.,0.,0.)) ;
#7047=DIRECTION('ref_axis',(0.,0.,-1.)) ;
#7048=DIRECTION('center_axis',(0.,1.,0.)) ;
#7049=DIRECTION('ref_axis',(0.,0.,1.)) ;
#7050=DIRECTION('center_axis',(0.,0.,-1.)) ;
#7051=DIRECTION('ref_axis',(-1.,0.,0.)) ;
#7052=DIRECTION('center_axis',(0.,1.,0.)) ;
#7053=DIRECTION('ref_axis',(-0.707106781186544,0.,-0.707106781186551)) ;
#7054=DIRECTION('center_axis',(0.,0.,1.)) ;
#7055=DIRECTION('ref_axis',(-0.707106781186552,0.707106781186543,0.)) ;
#7056=DIRECTION('',(0.,0.,1.)) ;
#7057=DIRECTION('center_axis',(0.,0.,-1.)) ;
#7058=DIRECTION('ref_axis',(-1.,0.,0.)) ;
#7059=DIRECTION('',(0.,1.,0.)) ;
#7060=DIRECTION('',(1.,0.,0.)) ;
#7061=DIRECTION('',(0.,1.,0.)) ;
#7062=DIRECTION('',(1.,0.,0.)) ;
#7063=DIRECTION('center_axis',(0.,1.,0.)) ;
#7064=DIRECTION('ref_axis',(1.,0.,-6.83214169000097E-15)) ;
#7065=DIRECTION('',(0.,1.,0.)) ;
#7066=DIRECTION('center_axis',(0.,1.,0.)) ;
#7067=DIRECTION('ref_axis',(1.,0.,-6.83214169000097E-15)) ;
#7068=DIRECTION('center_axis',(1.,0.,0.)) ;
#7069=DIRECTION('ref_axis',(0.,0.,-1.)) ;
#7070=DIRECTION('',(0.,1.,0.)) ;
#7071=DIRECTION('',(0.,0.,1.)) ;
#7072=DIRECTION('center_axis',(0.,1.,0.)) ;
#7073=DIRECTION('ref_axis',(0.427975386405345,0.,0.903790389764793)) ;
#7074=DIRECTION('',(0.,1.,0.)) ;
#7075=DIRECTION('center_axis',(0.,1.,0.)) ;
#7076=DIRECTION('ref_axis',(0.427975386405345,0.,0.903790389764793)) ;
#7077=DIRECTION('center_axis',(0.,1.,0.)) ;
#7078=DIRECTION('ref_axis',(-0.450036391082836,0.,0.893010216459552)) ;
#7079=DIRECTION('',(0.,1.,0.)) ;
#7080=DIRECTION('center_axis',(0.,1.,0.)) ;
#7081=DIRECTION('ref_axis',(-0.450036391082836,0.,0.893010216459552)) ;
#7082=DIRECTION('center_axis',(0.,1.,0.)) ;
#7083=DIRECTION('ref_axis',(-0.9998388850409,0.,0.0179500406732147)) ;
#7084=DIRECTION('',(0.,1.,0.)) ;
#7085=DIRECTION('center_axis',(0.,1.,0.)) ;
#7086=DIRECTION('ref_axis',(-0.9998388850409,0.,0.0179500406732147)) ;
#7087=DIRECTION('center_axis',(-1.,0.,0.)) ;
#7088=DIRECTION('ref_axis',(0.,0.,1.)) ;
#7089=DIRECTION('',(0.,1.,0.)) ;
#7090=DIRECTION('',(0.,0.,-1.)) ;
#7091=DIRECTION('center_axis',(0.,1.,0.)) ;
#7092=DIRECTION('ref_axis',(0.,0.,-1.)) ;
#7093=DIRECTION('',(0.,1.,0.)) ;
#7094=DIRECTION('center_axis',(0.,1.,0.)) ;
#7095=DIRECTION('ref_axis',(0.,0.,-1.)) ;
#7096=DIRECTION('center_axis',(0.,0.,-1.)) ;
#7097=DIRECTION('ref_axis',(-1.,0.,0.)) ;
#7098=DIRECTION('',(1.,0.,0.)) ;
#7099=DIRECTION('',(0.,-1.,0.)) ;
#7100=DIRECTION('',(1.,0.,0.)) ;
#7101=DIRECTION('center_axis',(1.,0.,0.)) ;
#7102=DIRECTION('ref_axis',(0.,0.,-1.)) ;
#7103=DIRECTION('',(1.,0.,0.)) ;
#7104=DIRECTION('center_axis',(-1.,0.,0.)) ;
#7105=DIRECTION('ref_axis',(0.,0.,-1.)) ;
#7106=DIRECTION('center_axis',(1.,0.,0.)) ;
#7107=DIRECTION('ref_axis',(0.,0.,-1.)) ;
#7108=DIRECTION('center_axis',(1.,0.,0.)) ;
#7109=DIRECTION('ref_axis',(0.,0.,-1.)) ;
#7110=DIRECTION('',(1.,0.,0.)) ;
#7111=DIRECTION('center_axis',(1.,0.,0.)) ;
#7112=DIRECTION('ref_axis',(0.,0.,-1.)) ;
#7113=DIRECTION('',(0.,0.,-1.)) ;
#7114=DIRECTION('',(0.,-1.,0.)) ;
#7115=DIRECTION('',(0.,0.,1.)) ;
#7116=DIRECTION('center_axis',(1.,0.,0.)) ;
#7117=DIRECTION('ref_axis',(0.,0.,-1.)) ;
#7118=DIRECTION('',(0.,-1.,0.)) ;
#7119=DIRECTION('center_axis',(1.,0.,0.)) ;
#7120=DIRECTION('ref_axis',(0.,0.00361481447269016,-0.999993466536821)) ;
#7121=DIRECTION('center_axis',(0.,0.,1.)) ;
#7122=DIRECTION('ref_axis',(0.,-1.,0.)) ;
#7123=DIRECTION('',(0.,-1.,0.)) ;
#7124=DIRECTION('',(1.,0.,0.)) ;
#7125=DIRECTION('',(1.,0.,0.)) ;
#7126=DIRECTION('center_axis',(0.,1.,0.)) ;
#7127=DIRECTION('ref_axis',(0.,0.,1.)) ;
#7128=DIRECTION('',(0.,0.,1.)) ;
#7129=DIRECTION('',(1.,0.,0.)) ;
#7130=DIRECTION('center_axis',(1.,0.,0.)) ;
#7131=DIRECTION('ref_axis',(0.,0.,-1.)) ;
#7132=DIRECTION('center_axis',(1.,0.,0.)) ;
#7133=DIRECTION('ref_axis',(0.,0.,-1.)) ;
#7134=DIRECTION('',(1.,0.,0.)) ;
#7135=DIRECTION('center_axis',(0.,0.,1.)) ;
#7136=DIRECTION('ref_axis',(0.,-1.,0.)) ;
#7137=DIRECTION('',(-1.,0.,0.)) ;
#7138=DIRECTION('',(0.,-1.,0.)) ;
#7139=DIRECTION('center_axis',(1.,0.,0.)) ;
#7140=DIRECTION('ref_axis',(0.,0.,-1.)) ;
#7141=DIRECTION('center_axis',(-1.,0.,0.)) ;
#7142=DIRECTION('ref_axis',(0.,0.00361481447269016,-0.999993466536821)) ;
#7143=DIRECTION('',(0.,0.,1.)) ;
#7144=DIRECTION('center_axis',(0.,1.,0.)) ;
#7145=DIRECTION('ref_axis',(1.,0.,0.)) ;
#7146=DIRECTION('',(-1.,0.,0.)) ;
#7147=DIRECTION('center_axis',(0.,-1.,0.)) ;
#7148=DIRECTION('ref_axis',(8.33188010975728E-16,0.,1.)) ;
#7149=DIRECTION('',(-1.,0.,0.)) ;
#7150=DIRECTION('center_axis',(0.,-1.,0.)) ;
#7151=DIRECTION('ref_axis',(8.33188010975728E-16,0.,1.)) ;
#7152=DIRECTION('center_axis',(0.,0.245126981107871,0.969490981460344)) ;
#7153=DIRECTION('ref_axis',(0.,-0.969490981460344,0.245126981107871)) ;
#7154=DIRECTION('',(1.,0.,0.)) ;
#7155=DIRECTION('center_axis',(1.,0.,0.)) ;
#7156=DIRECTION('ref_axis',(0.,0.00361481447269016,-0.999993466536821)) ;
#7157=DIRECTION('center_axis',(0.,0.,-1.)) ;
#7158=DIRECTION('ref_axis',(-1.,0.,0.)) ;
#7159=DIRECTION('',(0.,1.,0.)) ;
#7160=DIRECTION('center_axis',(0.,1.,0.)) ;
#7161=DIRECTION('ref_axis',(8.33188010975728E-16,0.,1.)) ;
#7162=DIRECTION('center_axis',(0.,0.,-1.)) ;
#7163=DIRECTION('ref_axis',(-1.,0.,0.)) ;
#7164=DIRECTION('',(0.,1.,0.)) ;
#7165=DIRECTION('center_axis',(0.,1.,0.)) ;
#7166=DIRECTION('ref_axis',(8.33188010975728E-16,0.,1.)) ;
#9094=CARTESIAN_POINT('',(0.,0.,0.)) ;
#9095=CARTESIAN_POINT('Origin',(-9.75,3.55,44.8475)) ;
#9096=CARTESIAN_POINT('',(-9.73166789581674,3.300673038048,52.4412514394322)) ;
#9097=CARTESIAN_POINT('',(-9.5,3.55,51.7196985577435)) ;
#9098=CARTESIAN_POINT('Ctrl Pts',(-9.73166789581674,3.300673038048,52.4412514394322)) ;
#9099=CARTESIAN_POINT('Ctrl Pts',(-9.72011624748849,3.30152238871182,52.4296997911002)) ;
#9100=CARTESIAN_POINT('Ctrl Pts',(-9.71077453059008,3.30297344738984,52.4127655658232)) ;
#9101=CARTESIAN_POINT('Ctrl Pts',(-9.66740696188674,3.31125291954623,52.3320464604663)) ;
#9102=CARTESIAN_POINT('Ctrl Pts',(-9.63485752215083,3.32587980802581,52.2484283731037)) ;
#9103=CARTESIAN_POINT('Ctrl Pts',(-9.58078548283598,3.3628440108946,52.104753223308)) ;
#9104=CARTESIAN_POINT('Ctrl Pts',(-9.55334337963797,3.39036468556239,52.0234232206868)) ;
#9105=CARTESIAN_POINT('Ctrl Pts',(-9.51285745751298,3.4610024800945,51.8649901763511)) ;
#9106=CARTESIAN_POINT('Ctrl Pts',(-9.5,3.50416452181587,51.7878595996225)) ;
#9107=CARTESIAN_POINT('Ctrl Pts',(-9.5,3.55,51.7196985577435)) ;
#9108=CARTESIAN_POINT('',(-9.5,3.55,35.75)) ;
#9109=CARTESIAN_POINT('',(-9.5,3.55,44.8475)) ;
#9110=CARTESIAN_POINT('',(-9.75,3.3,35.75)) ;
#9111=CARTESIAN_POINT('Origin',(-9.75,3.55,35.75)) ;
#9112=CARTESIAN_POINT('',(-9.75,3.3,52.4595835436154)) ;
#9113=CARTESIAN_POINT('',(-9.75,3.3,44.8475)) ;
#9114=CARTESIAN_POINT('Origin',(-9.75,3.55,52.4595835436154)) ;
#9115=CARTESIAN_POINT('Origin',(-9.75,3.05,35.75)) ;
#9116=CARTESIAN_POINT('',(-9.5,3.48301270189222,35.5)) ;
#9117=CARTESIAN_POINT('',(-9.75,3.05,35.5)) ;
#9118=CARTESIAN_POINT('Ctrl Pts',(-9.5,3.48301270189222,35.5)) ;
#9119=CARTESIAN_POINT('Ctrl Pts',(-9.5,3.41929334642333,35.5)) ;
#9120=CARTESIAN_POINT('Ctrl Pts',(-9.52239299997444,3.34618261828772,35.5)) ;
#9121=CARTESIAN_POINT('Ctrl Pts',(-9.59902182095282,3.203805818051,35.5)) ;
#9122=CARTESIAN_POINT('Ctrl Pts',(-9.68072544447976,3.11927455552024,35.5)) ;
#9123=CARTESIAN_POINT('Ctrl Pts',(-9.75,3.05,35.5)) ;
#9124=CARTESIAN_POINT('Origin',(-9.75,3.05,35.75)) ;
#9125=CARTESIAN_POINT('Origin',(-9.5,3.05,35.75)) ;
#9126=CARTESIAN_POINT('Origin',(-9.5,14.6475105520359,44.075)) ;
#9127=CARTESIAN_POINT('',(-9.5,4.45,51.1)) ;
#9128=CARTESIAN_POINT('Origin',(-9.5,4.78534007458122,52.5504136037216)) ;
#9129=CARTESIAN_POINT('',(-9.5,22.05,46.65)) ;
#9130=CARTESIAN_POINT('',(-9.5,22.05,46.65)) ;
#9131=CARTESIAN_POINT('',(-9.5,20.65,35.5)) ;
#9132=CARTESIAN_POINT('Origin',(-9.5,20.629520265574,41.1654638231566)) ;
#9133=CARTESIAN_POINT('',(-9.5,3.,35.5)) ;
#9134=CARTESIAN_POINT('',(-9.5,19.79,40.28)) ;
#9135=CARTESIAN_POINT('Origin',(-9.5,19.79,38.695)) ;
#9136=CARTESIAN_POINT('Origin',(9.75,3.05,35.75)) ;
#9137=CARTESIAN_POINT('',(9.5,3.55,35.75)) ;
#9138=CARTESIAN_POINT('',(9.75,3.3,35.75)) ;
#9139=CARTESIAN_POINT('Origin',(9.75,3.55,35.75)) ;
#9140=CARTESIAN_POINT('',(9.75,3.05,35.5)) ;
#9141=CARTESIAN_POINT('Origin',(9.75,3.05,35.75)) ;
#9142=CARTESIAN_POINT('',(9.5,3.48301270189222,35.5)) ;
#9143=CARTESIAN_POINT('Ctrl Pts',(9.75,3.05,35.5)) ;
#9144=CARTESIAN_POINT('Ctrl Pts',(9.68072544447976,3.11927455552024,35.5)) ;
#9145=CARTESIAN_POINT('Ctrl Pts',(9.59902182095282,3.203805818051,35.5)) ;
#9146=CARTESIAN_POINT('Ctrl Pts',(9.52239299997444,3.34618261828772,35.5)) ;
#9147=CARTESIAN_POINT('Ctrl Pts',(9.5,3.41929334642333,35.5)) ;
#9148=CARTESIAN_POINT('Ctrl Pts',(9.5,3.48301270189222,35.5)) ;
#9149=CARTESIAN_POINT('Origin',(9.5,3.05,35.75)) ;
#9150=CARTESIAN_POINT('Origin',(9.75,3.55,44.8475)) ;
#9151=CARTESIAN_POINT('',(9.75,3.3,52.4595835436154)) ;
#9152=CARTESIAN_POINT('',(9.73166789577781,3.30067303805086,52.4412514393933)) ;
#9153=CARTESIAN_POINT('Origin',(9.75,3.55,52.4595835436154)) ;
#9154=CARTESIAN_POINT('',(9.75,3.3,44.8475)) ;
#9155=CARTESIAN_POINT('',(9.5,3.55,51.7196985577435)) ;
#9156=CARTESIAN_POINT('',(9.5,3.55,44.8475)) ;
#9157=CARTESIAN_POINT('Ctrl Pts',(9.5,3.55,51.7196985577435)) ;
#9158=CARTESIAN_POINT('Ctrl Pts',(9.5,3.50416452181587,51.7878595996225)) ;
#9159=CARTESIAN_POINT('Ctrl Pts',(9.51285745751298,3.4610024800945,51.8649901763511)) ;
#9160=CARTESIAN_POINT('Ctrl Pts',(9.55334337963797,3.39036468556239,52.0234232206868)) ;
#9161=CARTESIAN_POINT('Ctrl Pts',(9.58078548283598,3.3628440108946,52.104753223308)) ;
#9162=CARTESIAN_POINT('Ctrl Pts',(9.63485752215083,3.32587980802581,52.2484283731037)) ;
#9163=CARTESIAN_POINT('Ctrl Pts',(9.66740696188674,3.31125291954623,52.3320464604663)) ;
#9164=CARTESIAN_POINT('Ctrl Pts',(9.71077453058148,3.30297344739148,52.4127655658072)) ;
#9165=CARTESIAN_POINT('Ctrl Pts',(9.72011624746926,3.30152238871505,52.4296997910605)) ;
#9166=CARTESIAN_POINT('Ctrl Pts',(9.7316678957778,3.30067303805086,52.4412514393933)) ;
#9167=CARTESIAN_POINT('Origin',(9.5,14.6475105520359,44.075)) ;
#9168=CARTESIAN_POINT('',(9.5,20.65,35.5)) ;
#9169=CARTESIAN_POINT('',(9.5,3.,35.5)) ;
#9170=CARTESIAN_POINT('',(9.5,22.05,46.65)) ;
#9171=CARTESIAN_POINT('Origin',(9.5,20.629520265574,41.1654638231566)) ;
#9172=CARTESIAN_POINT('',(9.5,4.45,51.1)) ;
#9173=CARTESIAN_POINT('',(9.5,22.05,46.65)) ;
#9174=CARTESIAN_POINT('Origin',(9.5,4.78534007458122,52.5504136037216)) ;
#9175=CARTESIAN_POINT('',(9.5,19.79,40.28)) ;
#9176=CARTESIAN_POINT('Origin',(9.5,19.79,38.695)) ;
#9177=CARTESIAN_POINT('Origin',(-19.8,3.05,45.625)) ;
#9178=CARTESIAN_POINT('',(-19.8,3.3,48.54)) ;
#9179=CARTESIAN_POINT('',(-19.8,3.05,48.29)) ;
#9180=CARTESIAN_POINT('Origin',(-19.8,3.05,48.54)) ;
#9181=CARTESIAN_POINT('',(-19.8,3.05,42.96)) ;
#9182=CARTESIAN_POINT('Origin',(-19.8,3.05,45.625)) ;
#9183=CARTESIAN_POINT('',(-19.8,3.3,42.71)) ;
#9184=CARTESIAN_POINT('Origin',(-19.8,3.05,42.71)) ;
#9185=CARTESIAN_POINT('Origin',(-19.8,3.3,45.625)) ;
#9186=CARTESIAN_POINT('Origin',(-9.89996640571749,3.05,42.71)) ;
#9187=CARTESIAN_POINT('',(-16.75,3.05,42.96)) ;
#9188=CARTESIAN_POINT('',(-16.75,3.3,42.71)) ;
#9189=CARTESIAN_POINT('Origin',(-16.75,3.05,42.71)) ;
#9190=CARTESIAN_POINT('',(-9.89996640571749,3.3,42.71)) ;
#9191=CARTESIAN_POINT('',(-9.89996640571749,3.05,42.96)) ;
#9192=CARTESIAN_POINT('Origin',(-16.75,3.05,45.625)) ;
#9193=CARTESIAN_POINT('',(-16.75,3.05,48.29)) ;
#9194=CARTESIAN_POINT('',(-16.75,3.3,48.54)) ;
#9195=CARTESIAN_POINT('Origin',(-16.75,3.05,48.54)) ;
#9196=CARTESIAN_POINT('Origin',(-16.75,3.3,45.625)) ;
#9197=CARTESIAN_POINT('Origin',(-16.75,3.05,45.625)) ;
#9198=CARTESIAN_POINT('Origin',(-8.3749664057175,3.05,48.54)) ;
#9199=CARTESIAN_POINT('',(-8.3749664057175,3.3,48.54)) ;
#9200=CARTESIAN_POINT('',(-8.3749664057175,3.05,48.29)) ;
#9201=CARTESIAN_POINT('Origin',(-19.8,0.,42.96)) ;
#9202=CARTESIAN_POINT('',(-19.8,0.,42.96)) ;
#9203=CARTESIAN_POINT('',(-19.8,0.,42.96)) ;
#9204=CARTESIAN_POINT('',(-16.75,0.,42.96)) ;
#9205=CARTESIAN_POINT('',(-16.75,0.,42.96)) ;
#9206=CARTESIAN_POINT('',(-16.75,0.,42.96)) ;
#9207=CARTESIAN_POINT('Origin',(-19.8,0.,45.625)) ;
#9208=CARTESIAN_POINT('',(-19.8,0.,48.29)) ;
#9209=CARTESIAN_POINT('',(-19.8,0.,48.29)) ;
#9210=CARTESIAN_POINT('Origin',(-19.8,0.,45.625)) ;
#9211=CARTESIAN_POINT('Origin',(6.71885650094239E-5,3.3,45.62)) ;
#9212=CARTESIAN_POINT('',(-24.1,3.3,35.75)) ;
#9213=CARTESIAN_POINT('',(12.0500335942825,3.3,35.75)) ;
#9214=CARTESIAN_POINT('',(-24.5,3.3,36.15)) ;
#9215=CARTESIAN_POINT('Origin',(-24.1,3.3,36.15)) ;
#9216=CARTESIAN_POINT('',(-24.5,3.3,45.0477339100826)) ;
#9217=CARTESIAN_POINT('',(-24.5,3.3,40.885)) ;
#9218=CARTESIAN_POINT('',(-21.0874960519899,3.3,50.4767448507153)) ;
#9219=CARTESIAN_POINT('Origin',(-18.2944180372184,3.3,44.9341033685178)) ;
#9220=CARTESIAN_POINT('',(21.0902564701365,3.3,50.4753536112778)) ;
#9221=CARTESIAN_POINT('Origin',(0.,3.3,8.63269841269837)) ;
#9222=CARTESIAN_POINT('',(24.4999999432639,3.3,45.0508225837103)) ;
#9223=CARTESIAN_POINT('Origin',(18.5438728059353,3.3,45.0908404355877)) ;
#9224=CARTESIAN_POINT('',(24.5,3.3,36.15)) ;
#9225=CARTESIAN_POINT('',(24.5,3.3,45.335)) ;
#9226=CARTESIAN_POINT('',(24.1,3.3,35.75)) ;
#9227=CARTESIAN_POINT('Origin',(24.1,3.3,36.15)) ;
#9228=CARTESIAN_POINT('',(12.0500335942825,3.3,35.75)) ;
#9229=CARTESIAN_POINT('',(-9.5,3.3,52.4595835436154)) ;
#9230=CARTESIAN_POINT('',(16.75,3.3,42.71)) ;
#9231=CARTESIAN_POINT('',(16.75,3.3,48.54)) ;
#9232=CARTESIAN_POINT('Origin',(16.75,3.3,45.625)) ;
#9233=CARTESIAN_POINT('',(19.8,3.3,42.71)) ;
#9234=CARTESIAN_POINT('',(8.3750335942825,3.3,42.71)) ;
#9235=CARTESIAN_POINT('',(19.8,3.3,48.54)) ;
#9236=CARTESIAN_POINT('Origin',(19.8,3.3,45.625)) ;
#9237=CARTESIAN_POINT('',(9.9000335942825,3.3,48.54)) ;
#9238=CARTESIAN_POINT('Origin',(16.75,3.05,45.625)) ;
#9239=CARTESIAN_POINT('',(16.75,3.05,48.29)) ;
#9240=CARTESIAN_POINT('Origin',(16.75,3.05,48.54)) ;
#9241=CARTESIAN_POINT('',(16.75,3.05,42.96)) ;
#9242=CARTESIAN_POINT('Origin',(16.75,3.05,45.625)) ;
#9243=CARTESIAN_POINT('Origin',(16.75,3.05,42.71)) ;
#9244=CARTESIAN_POINT('Origin',(8.3750335942825,3.05,42.71)) ;
#9245=CARTESIAN_POINT('',(19.8,3.05,42.96)) ;
#9246=CARTESIAN_POINT('Origin',(19.8,3.05,42.71)) ;
#9247=CARTESIAN_POINT('',(8.3750335942825,3.05,42.96)) ;
#9248=CARTESIAN_POINT('Origin',(19.8,3.05,45.625)) ;
#9249=CARTESIAN_POINT('',(19.8,3.05,48.29)) ;
#9250=CARTESIAN_POINT('Origin',(19.8,3.05,48.54)) ;
#9251=CARTESIAN_POINT('Origin',(19.8,3.05,45.625)) ;
#9252=CARTESIAN_POINT('Origin',(9.9000335942825,3.05,48.54)) ;
#9253=CARTESIAN_POINT('',(9.9000335942825,3.05,48.29)) ;
#9254=CARTESIAN_POINT('Origin',(16.75,0.,42.96)) ;
#9255=CARTESIAN_POINT('',(16.75,0.,42.96)) ;
#9256=CARTESIAN_POINT('',(16.75,0.,42.96)) ;
#9257=CARTESIAN_POINT('',(19.8,0.,42.96)) ;
#9258=CARTESIAN_POINT('',(19.8,0.,42.96)) ;
#9259=CARTESIAN_POINT('',(19.8,0.,42.96)) ;
#9260=CARTESIAN_POINT('Origin',(16.75,0.,45.625)) ;
#9261=CARTESIAN_POINT('',(16.75,0.,48.29)) ;
#9262=CARTESIAN_POINT('',(16.75,0.,48.29)) ;
#9263=CARTESIAN_POINT('Origin',(16.75,0.,45.625)) ;
#9264=CARTESIAN_POINT('Origin',(-9.5,3.55,52.4595835436154)) ;
#9265=CARTESIAN_POINT('',(-9.5,3.30067303804748,52.4412514394393)) ;
#9266=CARTESIAN_POINT('Origin',(-9.5,4.78534007458122,52.5504136037216)) ;
#9267=CARTESIAN_POINT('',(-9.5,4.45,51.1)) ;
#9268=CARTESIAN_POINT('Origin',(18.5438728059353,3.05,45.0908404355877)) ;
#9269=CARTESIAN_POINT('',(21.2,3.05,50.7)) ;
#9270=CARTESIAN_POINT('',(24.75,3.05,45.05)) ;
#9271=CARTESIAN_POINT('Origin',(18.5438728059353,3.05,45.0908404355877)) ;
#9272=CARTESIAN_POINT('Ctrl Pts',(24.75,3.05,45.05)) ;
#9273=CARTESIAN_POINT('Ctrl Pts',(24.7499997649959,3.06636246173745,45.0499642886908)) ;
#9274=CARTESIAN_POINT('Ctrl Pts',(24.7483880426071,3.08272451888078,45.0499391822158)) ;
#9275=CARTESIAN_POINT('Ctrl Pts',(24.7451957187188,3.09877258050403,45.049924559718)) ;
#9276=CARTESIAN_POINT('Ctrl Pts',(24.742135735277,3.11415535636217,45.0499105434081)) ;
#9277=CARTESIAN_POINT('Ctrl Pts',(24.7376239954586,3.12924901976136,45.049906156751)) ;
#9278=CARTESIAN_POINT('Ctrl Pts',(24.7317399828519,3.14378765298013,45.0499109447592)) ;
#9279=CARTESIAN_POINT('Ctrl Pts',(24.7258570786838,3.15832354739046,45.0499157318653)) ;
#9280=CARTESIAN_POINT('Ctrl Pts',(24.7186026657308,3.17230401465796,45.0499296888126)) ;
#9281=CARTESIAN_POINT('Ctrl Pts',(24.7101044996307,3.18548284147049,45.0499520344104)) ;
#9282=CARTESIAN_POINT('Ctrl Pts',(24.7016076986088,3.19865955134022,45.0499743764187)) ;
#9283=CARTESIAN_POINT('Ctrl Pts',(24.6918678995193,3.211034329459,45.0500051022664)) ;
#9284=CARTESIAN_POINT('Ctrl Pts',(24.6810565738722,3.22238931032504,45.0500431309344)) ;
#9285=CARTESIAN_POINT('Ctrl Pts',(24.6702466852255,3.23374278193012,45.0500811545477)) ;
#9286=CARTESIAN_POINT('Ctrl Pts',(24.6583660062662,3.24407625489886,45.0501264762469)) ;
#9287=CARTESIAN_POINT('Ctrl Pts',(24.6456236446434,3.25320785025283,45.0501777521907)) ;
#9288=CARTESIAN_POINT('Ctrl Pts',(24.6328768472724,3.26234262440984,45.0502290459843)) ;
#9289=CARTESIAN_POINT('Ctrl Pts',(24.6192682971389,3.27027430056404,45.0502862948054)) ;
#9290=CARTESIAN_POINT('Ctrl Pts',(24.6050376799198,3.27686317695211,45.0503479362075)) ;
#9291=CARTESIAN_POINT('Ctrl Pts',(24.5908114805106,3.28345000786299,45.0504095584734)) ;
#9292=CARTESIAN_POINT('Ctrl Pts',(24.575964194553,3.28869460036439,45.0504755667426)) ;
#9293=CARTESIAN_POINT('Ctrl Pts',(24.5607571642129,3.29250463772944,45.050544237254)) ;
#9294=CARTESIAN_POINT('Ctrl Pts',(24.5455488731175,3.29631499096976,45.0506129134587)) ;
#9295=CARTESIAN_POINT('Ctrl Pts',(24.5299814118393,3.29869039164851,45.0506842481721)) ;
#9296=CARTESIAN_POINT('Ctrl Pts',(24.5143288443927,3.29958902042781,45.0507564146933)) ;
#9297=CARTESIAN_POINT('Ctrl Pts',(24.5095577809545,3.29986293171604,45.0507784117907)) ;
#9298=CARTESIAN_POINT('Ctrl Pts',(24.5047788624715,3.3,45.0508004856938)) ;
#9299=CARTESIAN_POINT('Ctrl Pts',(24.4999999432639,3.3,45.0508225837103)) ;
#9300=CARTESIAN_POINT('Ctrl Pts',(21.0902564701365,3.3,50.4753536112778)) ;
#9301=CARTESIAN_POINT('Ctrl Pts',(21.0907463180989,3.3,50.4763566221903)) ;
#9302=CARTESIAN_POINT('Ctrl Pts',(21.09123616212,3.29999252528887,50.4773596211075)) ;
#9303=CARTESIAN_POINT('Ctrl Pts',(21.1060035602585,3.29954182407199,50.5075970557322)) ;
#9304=CARTESIAN_POINT('Ctrl Pts',(21.1201089113617,3.29275962387286,50.5364754558814)) ;
#9305=CARTESIAN_POINT('Ctrl Pts',(21.1463954963948,3.26725755617282,50.5902876319832)) ;
#9306=CARTESIAN_POINT('Ctrl Pts',(21.1583244312364,3.24877490065223,50.6147049771605)) ;
#9307=CARTESIAN_POINT('Ctrl Pts',(21.1784011784248,3.20243491264089,50.6557973965193)) ;
#9308=CARTESIAN_POINT('Ctrl Pts',(21.1863573189541,3.17502132423592,50.6720802410836)) ;
#9309=CARTESIAN_POINT('Ctrl Pts',(21.1972085288292,3.11479146985681,50.6942875251967)) ;
#9310=CARTESIAN_POINT('Ctrl Pts',(21.1999999999996,3.0825514085482,50.7000000000002)) ;
#9311=CARTESIAN_POINT('Ctrl Pts',(21.1999999999996,3.05,50.7000000000002)) ;
#9312=CARTESIAN_POINT('Origin',(24.5,3.05,45.335)) ;
#9313=CARTESIAN_POINT('',(24.75,3.05,36.15)) ;
#9314=CARTESIAN_POINT('',(24.75,3.05,45.335)) ;
#9315=CARTESIAN_POINT('Origin',(24.5,3.05,36.15)) ;
#9316=CARTESIAN_POINT('Origin',(24.1,3.05,36.15)) ;
#9317=CARTESIAN_POINT('',(24.1,3.05,35.5)) ;
#9318=CARTESIAN_POINT('Origin',(24.1,3.05,35.75)) ;
#9319=CARTESIAN_POINT('Origin',(24.1,3.05,36.15)) ;
#9320=CARTESIAN_POINT('Origin',(12.0500335942825,3.05,35.75)) ;
#9321=CARTESIAN_POINT('',(12.0500335942825,3.05,35.5)) ;
#9322=CARTESIAN_POINT('Origin',(-18.2944180372184,3.05,44.9341033685178)) ;
#9323=CARTESIAN_POINT('',(-24.75,3.05,45.05)) ;
#9324=CARTESIAN_POINT('',(-21.2,3.05,50.7)) ;
#9325=CARTESIAN_POINT('Origin',(-18.2944180372184,3.05,44.9341033685178)) ;
#9326=CARTESIAN_POINT('Origin',(-21.0874960519899,3.05,50.4767448507153)) ;
#9327=CARTESIAN_POINT('Ctrl Pts',(-24.5,3.3,45.0477339100826)) ;
#9328=CARTESIAN_POINT('Ctrl Pts',(-24.5012372116335,3.3,45.0477452364374)) ;
#9329=CARTESIAN_POINT('Ctrl Pts',(-24.5024744062464,3.29999081584422,45.0477565609417)) ;
#9330=CARTESIAN_POINT('Ctrl Pts',(-24.5361188401082,3.29949127800647,45.048064475043)) ;
#9331=CARTESIAN_POINT('Ctrl Pts',(-24.5681256225385,3.29271255013592,45.0483562015273)) ;
#9332=CARTESIAN_POINT('Ctrl Pts',(-24.6278967898402,3.26726052961233,45.04889912374)) ;
#9333=CARTESIAN_POINT('Ctrl Pts',(-24.6550706061608,3.24877842887715,45.0491449678964)) ;
#9334=CARTESIAN_POINT('Ctrl Pts',(-24.7008035019926,3.2024389100284,45.0495577649017)) ;
#9335=CARTESIAN_POINT('Ctrl Pts',(-24.7189257200146,3.17502490071193,45.0497208021766)) ;
#9336=CARTESIAN_POINT('Ctrl Pts',(-24.7436420186525,3.11479366304012,45.0499429715952)) ;
#9337=CARTESIAN_POINT('Ctrl Pts',(-24.75,3.08255247821287,45.05)) ;
#9338=CARTESIAN_POINT('Ctrl Pts',(-24.75,3.05,45.05)) ;
#9339=CARTESIAN_POINT('Origin',(0.,3.05,8.63269841269837)) ;
#9340=CARTESIAN_POINT('Origin',(0.,3.05,8.63269841269837)) ;
#9341=CARTESIAN_POINT('Origin',(12.0500335942825,3.05,35.75)) ;
#9342=CARTESIAN_POINT('',(-24.1,3.05,35.5)) ;
#9343=CARTESIAN_POINT('',(12.0500335942825,3.05,35.5)) ;
#9344=CARTESIAN_POINT('Origin',(-24.1,3.05,35.75)) ;
#9345=CARTESIAN_POINT('Origin',(-24.1,3.05,36.15)) ;
#9346=CARTESIAN_POINT('',(-24.75,3.05,36.15)) ;
#9347=CARTESIAN_POINT('Origin',(-24.5,3.05,36.15)) ;
#9348=CARTESIAN_POINT('Origin',(-24.1,3.05,36.15)) ;
#9349=CARTESIAN_POINT('Origin',(-24.5,3.05,40.885)) ;
#9350=CARTESIAN_POINT('',(-24.75,3.05,40.885)) ;
#9351=CARTESIAN_POINT('Origin',(24.1,0.,35.5)) ;
#9352=CARTESIAN_POINT('',(24.1,0.,35.5)) ;
#9353=CARTESIAN_POINT('',(24.1,0.,35.5)) ;
#9354=CARTESIAN_POINT('',(6.95,0.,35.5)) ;
#9355=CARTESIAN_POINT('',(-24.1,0.,35.5)) ;
#9356=CARTESIAN_POINT('',(6.95,20.65,35.5)) ;
#9357=CARTESIAN_POINT('',(6.95,7.5,35.5)) ;
#9358=CARTESIAN_POINT('',(-9.5,20.65,35.5)) ;
#9359=CARTESIAN_POINT('Origin',(24.1,0.,36.15)) ;
#9360=CARTESIAN_POINT('',(24.75,0.,36.15)) ;
#9361=CARTESIAN_POINT('',(24.75,0.,36.15)) ;
#9362=CARTESIAN_POINT('Origin',(24.1,0.,36.15)) ;
#9363=CARTESIAN_POINT('Origin',(24.75,0.,45.05)) ;
#9364=CARTESIAN_POINT('',(24.75,0.,45.05)) ;
#9365=CARTESIAN_POINT('',(24.75,0.,45.05)) ;
#9366=CARTESIAN_POINT('',(24.75,0.,36.15)) ;
#9367=CARTESIAN_POINT('Origin',(18.5438728059353,0.,45.0908404355877)) ;
#9368=CARTESIAN_POINT('',(21.2,0.,50.7)) ;
#9369=CARTESIAN_POINT('',(21.2,0.,50.7)) ;
#9370=CARTESIAN_POINT('Origin',(18.5438728059353,0.,45.0908404355877)) ;
#9371=CARTESIAN_POINT('Origin',(0.,0.,8.63269841269837)) ;
#9372=CARTESIAN_POINT('',(-21.2,0.,50.7)) ;
#9373=CARTESIAN_POINT('',(-21.2,0.,50.7)) ;
#9374=CARTESIAN_POINT('Origin',(0.,0.,8.63269841269837)) ;
#9375=CARTESIAN_POINT('Origin',(-18.2944180372184,0.,44.9341033685178)) ;
#9376=CARTESIAN_POINT('',(-24.75,0.,45.05)) ;
#9377=CARTESIAN_POINT('',(-24.75,0.,45.05)) ;
#9378=CARTESIAN_POINT('Origin',(-18.2944180372184,0.,44.9341033685178)) ;
#9379=CARTESIAN_POINT('Origin',(-24.75,0.,36.15)) ;
#9380=CARTESIAN_POINT('',(-24.75,0.,36.15)) ;
#9381=CARTESIAN_POINT('',(-24.75,0.,36.15)) ;
#9382=CARTESIAN_POINT('',(-24.75,0.,45.05)) ;
#9383=CARTESIAN_POINT('Origin',(-24.1,0.,36.15)) ;
#9384=CARTESIAN_POINT('',(-24.1,0.,35.5)) ;
#9385=CARTESIAN_POINT('',(-24.1,0.,35.5)) ;
#9386=CARTESIAN_POINT('Origin',(-24.1,0.,36.15)) ;
#9387=CARTESIAN_POINT('Origin',(24.1,0.,35.5)) ;
#9388=CARTESIAN_POINT('',(-6.95,20.65,35.5)) ;
#9389=CARTESIAN_POINT('',(-9.5,20.65,35.5)) ;
#9390=CARTESIAN_POINT('',(-6.95,0.,35.5)) ;
#9391=CARTESIAN_POINT('',(-6.95,7.5,35.5)) ;
#9392=CARTESIAN_POINT('',(-24.1,0.,35.5)) ;
#9393=CARTESIAN_POINT('Origin',(-10.,19.79,38.695)) ;
#9394=CARTESIAN_POINT('',(-6.95,19.79,40.28)) ;
#9395=CARTESIAN_POINT('',(-10.,19.79,40.28)) ;
#9396=CARTESIAN_POINT('Origin',(-6.95,19.79,38.695)) ;
#9397=CARTESIAN_POINT('Origin',(-10.,19.79,38.695)) ;
#9398=CARTESIAN_POINT('',(6.95,19.79,40.28)) ;
#9399=CARTESIAN_POINT('Origin',(6.95,19.79,38.695)) ;
#9400=CARTESIAN_POINT('',(-10.,19.79,40.28)) ;
#9401=CARTESIAN_POINT('Origin',(6.95,15.,39.2475)) ;
#9402=CARTESIAN_POINT('',(6.95,0.,45.25)) ;
#9403=CARTESIAN_POINT('',(6.95,0.,42.43375)) ;
#9404=CARTESIAN_POINT('',(6.95,20.,45.25)) ;
#9405=CARTESIAN_POINT('',(6.95,20.,45.25)) ;
#9406=CARTESIAN_POINT('',(6.95,20.,44.1409526255743)) ;
#9407=CARTESIAN_POINT('',(6.95,20.,40.3)) ;
#9408=CARTESIAN_POINT('',(6.95,24.9983082666063,40.3)) ;
#9409=CARTESIAN_POINT('Origin',(6.95,19.79,38.695)) ;
#9410=CARTESIAN_POINT('',(6.95,26.2285266168675,40.3)) ;
#9411=CARTESIAN_POINT('',(6.95,30.,40.3)) ;
#9412=CARTESIAN_POINT('Origin',(6.95,20.629520265574,41.1654638231566)) ;
#9413=CARTESIAN_POINT('Origin',(-6.95,20.,45.25)) ;
#9414=CARTESIAN_POINT('',(-6.95,20.,45.25)) ;
#9415=CARTESIAN_POINT('',(-6.95,0.,45.25)) ;
#9416=CARTESIAN_POINT('',(-6.95,20.,45.25)) ;
#9417=CARTESIAN_POINT('',(-6.95,20.,45.25)) ;
#9418=CARTESIAN_POINT('',(-3.4749664057175,0.,45.25)) ;
#9419=CARTESIAN_POINT('Origin',(-6.95,20.,44.1409526255743)) ;
#9420=CARTESIAN_POINT('',(-6.95,20.,44.1409526255743)) ;
#9421=CARTESIAN_POINT('',(-6.95,20.,40.3)) ;
#9422=CARTESIAN_POINT('',(-6.95,20.,44.1409526255743)) ;
#9423=CARTESIAN_POINT('Origin',(-6.95,19.79,38.695)) ;
#9424=CARTESIAN_POINT('',(-6.95,24.9983082666063,40.3)) ;
#9425=CARTESIAN_POINT('Origin',(-6.95,19.79,38.695)) ;
#9426=CARTESIAN_POINT('',(-6.95,24.9983082666063,40.3)) ;
#9427=CARTESIAN_POINT('Origin',(-6.95,30.,40.3)) ;
#9428=CARTESIAN_POINT('',(-6.95,26.2285266168675,40.3)) ;
#9429=CARTESIAN_POINT('',(-9.5,26.2285266168675,40.3)) ;
#9430=CARTESIAN_POINT('',(-6.95,30.,40.3)) ;
#9431=CARTESIAN_POINT('Origin',(-6.95,15.,39.2475)) ;
#9432=CARTESIAN_POINT('Origin',(-6.95,20.629520265574,41.1654638231566)) ;
#9433=CARTESIAN_POINT('',(-6.95,0.,42.43375)) ;
#9434=CARTESIAN_POINT('Origin',(6.71885650094239E-5,0.,45.62)) ;
#9435=CARTESIAN_POINT('',(19.8,0.,48.29)) ;
#9436=CARTESIAN_POINT('',(16.75,0.,48.29)) ;
#9437=CARTESIAN_POINT('Origin',(19.8,0.,45.625)) ;
#9438=CARTESIAN_POINT('',(-16.75,0.,48.29)) ;
#9439=CARTESIAN_POINT('',(-19.8,0.,48.29)) ;
#9440=CARTESIAN_POINT('Origin',(-16.75,0.,45.625)) ;
#9441=CARTESIAN_POINT('Origin',(-9.5,22.05,46.65)) ;
#9442=CARTESIAN_POINT('',(-9.5,22.05,46.65)) ;
#9443=CARTESIAN_POINT('Origin',(-9.5,20.629520265574,41.1654638231566)) ;
#9444=CARTESIAN_POINT('Origin',(19.8,0.,48.29)) ;
#9445=CARTESIAN_POINT('',(19.8,0.,48.29)) ;
#9446=CARTESIAN_POINT('Origin',(19.8,0.,45.625)) ;
#9447=CARTESIAN_POINT('Origin',(-16.75,0.,48.29)) ;
#9448=CARTESIAN_POINT('',(-16.75,0.,48.29)) ;
#9449=CARTESIAN_POINT('Origin',(-16.75,0.,45.625)) ;
#11365=UNCERTAINTY_MEASURE_WITH_UNIT(LENGTH_MEASURE(0.01),#11397,
'DISTANCE_ACCURACY_VALUE',
'Maximum model space distance between geometric entities at asserted c
onnectivities') ;
#11379=UNCERTAINTY_MEASURE_WITH_UNIT(LENGTH_MEASURE(0.01),#11397,
'DISTANCE_ACCURACY_VALUE',
'Maximum model space distance between geometric entities at asserted c
onnectivities') ;
#11382=(
GEOMETRIC_REPRESENTATION_CONTEXT(3)
GLOBAL_UNCERTAINTY_ASSIGNED_CONTEXT((#11365))
GLOBAL_UNIT_ASSIGNED_CONTEXT((#11397,#11399,#11400))
REPRESENTATION_CONTEXT('','3D')
) ;
#11396=(
GEOMETRIC_REPRESENTATION_CONTEXT(3)
GLOBAL_UNCERTAINTY_ASSIGNED_CONTEXT((#11379))
GLOBAL_UNIT_ASSIGNED_CONTEXT((#11397,#11399,#11400))
REPRESENTATION_CONTEXT('','3D')
) ;
#11397=(
LENGTH_UNIT()
NAMED_UNIT(*)
SI_UNIT(.MILLI.,.METRE.)
) ;
#11399=(
NAMED_UNIT(*)
PLANE_ANGLE_UNIT()
SI_UNIT($,.RADIAN.)
) ;
#11400=(
NAMED_UNIT(*)
SI_UNIT($,.STERADIAN.)
SOLID_ANGLE_UNIT()
) ;
#11403=SHAPE_DEFINITION_REPRESENTATION(#11419,#11456) ;
#11419=PRODUCT_DEFINITION_SHAPE('',$,#11473) ;
#11456=SHAPE_REPRESENTATION('',(#5923),#11382) ;
#11470=PRODUCT_DEFINITION_CONTEXT('part definition',#11520,'design') ;
#11473=PRODUCT_DEFINITION('Strike Plate with Roller Ears',
'Strike Plate with Roller Ears',#11489,#11470) ;
#11489=PRODUCT_DEFINITION_FORMATION('',$,#11524) ;
#11520=APPLICATION_CONTEXT(
'Core Data for Automotive Mechanical Design Process') ;
#11521=PRODUCT_CONTEXT('part definition',#11520,'mechanical') ;
#11524=PRODUCT('Strike Plate with Roller Ears',
'Strike Plate with Roller Ears',$,(#11521)) ;
#11540=PRESENTATION_STYLE_ASSIGNMENT((#11556)) ;
#11556=SURFACE_STYLE_USAGE(.BOTH.,#11572) ;
#11572=SURFACE_SIDE_STYLE('',(#11588)) ;
#11588=SURFACE_STYLE_FILL_AREA(#11604) ;
#11604=FILL_AREA_STYLE(
'MAS-252 Grey Paint - Strike Plate with Roller Ears',(#11620)) ;
#11620=FILL_AREA_STYLE_COLOUR(
'MAS-252 Grey Paint - Strike Plate with Roller Ears',#11636) ;
#11636=COLOUR_RGB('MAS-252 Grey Paint - Strike Plate with Roller Ears', 0.66274510, 0.83137255, 0.94901961) ;
ENDSEC;
END-ISO-10303-21;
